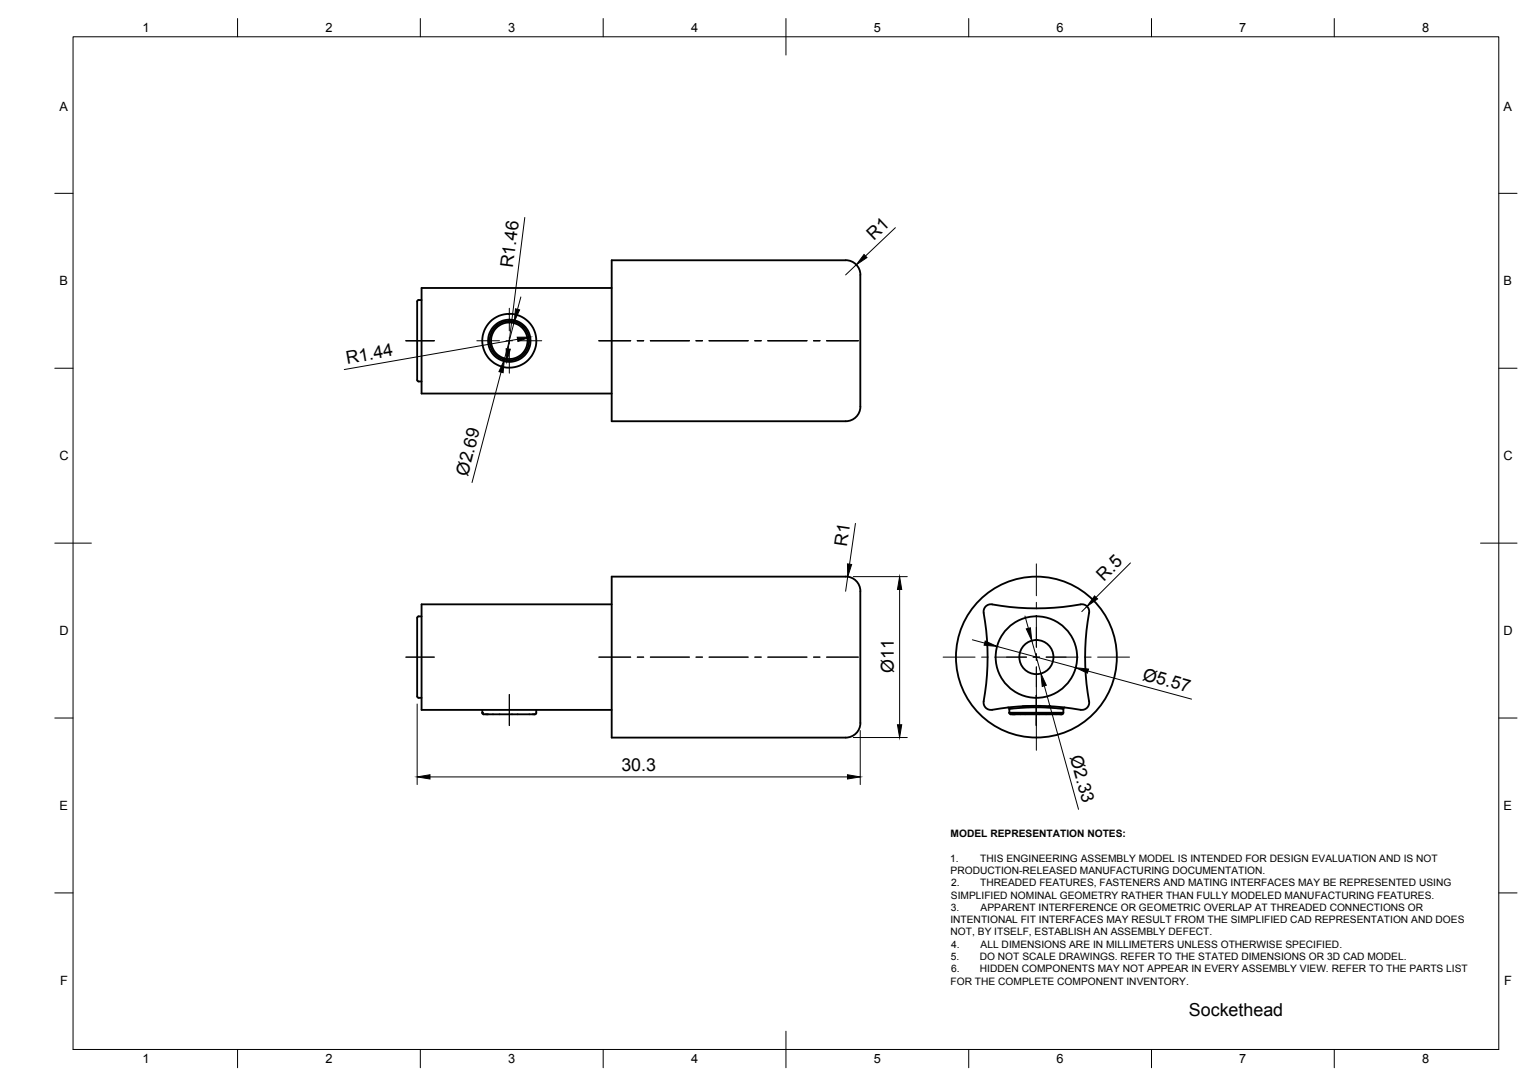
ISO-10303-21;
HEADER;
/* Generated by software containing ST-Developer
 * from STEP Tools, Inc. (www.steptools.com) 
 */

FILE_DESCRIPTION(
/* description */ ('STEP AP242 Edition 2'),
/* implementation_level */ '2;1');

FILE_NAME(
/* name */ 'Sockethead.step',
/* time_stamp */ '2026-10-06T10:11:12-07:00',
/* author */ (''),
/* organization */ (''),
/* preprocessor_version */ 'ST-DEVELOPER v20.2',
/* originating_system */ 'Autodesk Translation Framework v15.15.0.0',
/* authorisation */ '');

FILE_SCHEMA (('AUTOMOTIVE_DESIGN { 1 0 10303 214 3 1 1 }'));
ENDSEC;

DATA;
#10=MECHANICAL_DESIGN_GEOMETRIC_PRESENTATION_REPRESENTATION('',(#1787,#1788,#1789,#1790,#1791),#54580);
#235=TOROIDAL_SURFACE('',#18788,0.00268445714771808,0.0001);
#236=TOROIDAL_SURFACE('',#18804,0.00144581322131978,0.000100021493280238);
#237=TOROIDAL_SURFACE('',#18806,0.00106635989804114,0.0001);
#238=TOROIDAL_SURFACE('',#18808,0.00126635989804114,0.0001);
#239=TOROIDAL_SURFACE('',#18810,0.0045,0.001);
#1314=B_SPLINE_CURVE_WITH_KNOTS('',3,(#47239,#47240,#47241,#47242,#47243,
#47244,#47245,#47246,#47247,#47248,#47249),.UNSPECIFIED.,.F.,.F.,(4,1,1,
1,1,1,1,1,4),(3.17007800203674E-7,0.00137241382077849,0.00274482764155697,
0.00411724146233546,0.00548965528311394,0.00686206910389242,0.00823448292467091,
0.00960689674544939,0.0108038290876045),.UNSPECIFIED.);
#1315=B_SPLINE_CURVE_WITH_KNOTS('',3,(#47255,#47256,#47257,#47258,#47259,
#47260,#47261,#47262,#47263,#47264,#47265,#47266,#47267,#47268,#47269,#47270),
 .UNSPECIFIED.,.F.,.F.,(4,3,3,3,3,4),(0.5,0.51594481978154,0.641195140394408,
0.766134114390843,0.890913197743559,1.),.UNSPECIFIED.);
#1316=B_SPLINE_CURVE_WITH_KNOTS('',3,(#47271,#47272,#47273,#47274,#47275,
#47276,#47277,#47278,#47279,#47280,#47281,#47282,#47283),.UNSPECIFIED.,
 .F.,.F.,(4,3,3,3,4),(0.01606865131382,0.141192218026199,0.265882467388624,
0.390722415283828,0.5),.UNSPECIFIED.);
#1317=B_SPLINE_CURVE_WITH_KNOTS('',3,(#47323,#47324,#47325,#47326,#47327,
#47328,#47329,#47330,#47331,#47332,#47333,#47334,#47335),.UNSPECIFIED.,
 .F.,.F.,(4,3,3,3,4),(0.844373201093006,0.868421052636719,0.901315789477539,
0.934210526318359,0.956585831262424),.UNSPECIFIED.);
#1318=B_SPLINE_CURVE_WITH_KNOTS('',3,(#47337,#47338,#47339,#47340,#47341,
#47342,#47343,#47344,#47345,#47346,#47347,#47348,#47349,#47350,#47351,#47352,
#47353,#47354,#47355,#47356,#47357,#47358),.UNSPECIFIED.,.F.,.F.,(4,3,3,
3,3,3,3,4),(0.595152011141008,0.6184210546875,0.649671054199219,0.680921053710937,
0.743421052734375,0.774671052709961,0.805921052685547,0.844373201093006),
 .UNSPECIFIED.);
#1319=B_SPLINE_CURVE_WITH_KNOTS('',3,(#47360,#47361,#47362,#47363,#47364,
#47365,#47366,#47367,#47368,#47369),.UNSPECIFIED.,.F.,.F.,(4,3,3,4),(0.499571204578003,
0.524671083984375,0.55592107421875,0.595152011141008),.UNSPECIFIED.);
#1320=B_SPLINE_CURVE_WITH_KNOTS('',3,(#47371,#47372,#47373,#47374,#47375,
#47376,#47377,#47378,#47379,#47380,#47381,#47382,#47383,#47384,#47385,#47386),
 .UNSPECIFIED.,.F.,.F.,(4,3,3,3,3,4),(0.344377029418945,0.368421875,0.3996716796875,
0.430921484375,0.49342109375,0.499571204578003),.UNSPECIFIED.);
#1321=B_SPLINE_CURVE_WITH_KNOTS('',3,(#47388,#47389,#47390,#47391,#47392,
#47393,#47394,#47395,#47396,#47397,#47398,#47399,#47400,#47401,#47402,#47403,
#47404,#47405,#47406,#47407,#47408,#47409),.UNSPECIFIED.,.F.,.F.,(4,3,3,
3,3,3,3,4),(0.0951513536663715,0.11875,0.149921875,0.18109375,0.2434375,
0.27468359375,0.3059296875,0.344377029418945),.UNSPECIFIED.);
#1322=B_SPLINE_CURVE_WITH_KNOTS('',3,(#47411,#47412,#47413,#47414,#47415,
#47416,#47417),.UNSPECIFIED.,.F.,.F.,(4,3,4),(0.,0.059375,0.0951513536663715),
 .UNSPECIFIED.);
#1323=B_SPLINE_CURVE_WITH_KNOTS('',3,(#47422,#47423,#47424,#47425,#47426,
#47427,#47428,#47429,#47430,#47431,#47432,#47433,#47434,#47435,#47436,#47437,
#47438,#47439,#47440,#47441,#47442,#47443,#47444,#47445,#47446,#47447,#47448,
#47449),.UNSPECIFIED.,.F.,.F.,(4,3,3,3,3,3,3,3,3,4),(0.000439637419233018,
0.00197475622652821,0.00351361546357811,0.00505249384731604,0.00658820808674074,
0.00812412382728726,0.00966469812314125,0.0112015348521649,0.0122952440085163,
0.0122953616167891),.UNSPECIFIED.);
#1324=B_SPLINE_CURVE_WITH_KNOTS('',3,(#47498,#47499,#47500,#47501,#47502,
#47503,#47504,#47505,#47506,#47507,#47508,#47509,#47510,#47511,#47512,#47513,
#47514,#47515),.UNSPECIFIED.,.F.,.F.,(4,2,2,2,2,2,2,2,4),(0.0531545443972438,
0.0539804531362699,0.0553833366067717,0.063256430848433,0.0837219286225868,
0.0893954400242927,0.0917963407013744,0.109557936372639,0.132545890778438),
 .UNSPECIFIED.);
#1325=B_SPLINE_CURVE_WITH_KNOTS('',3,(#47519,#47520,#47521,#47522,#47523,
#47524,#47525,#47526,#47527,#47528,#47529,#47530,#47531,#47532,#47533,#47534,
#47535,#47536,#47537,#47538),.UNSPECIFIED.,.F.,.F.,(4,2,2,2,2,2,2,2,2,4),
(-0.158319955435896,-0.133815137850197,-0.106658138126813,-0.1025999008806,
-0.10032932226052,-0.0927408284757264,-0.079200925255067,-0.0410108789329117,
-0.0204087370161667,-3.15727931039809E-5),.UNSPECIFIED.);
#1326=B_SPLINE_CURVE_WITH_KNOTS('',3,(#47540,#47541,#47542,#47543,#47544,
#47545,#47546,#47547,#47548,#47549,#47550,#47551,#47552,#47553,#47554,#47555,
#47556,#47557,#47558,#47559,#47560,#47561,#47562,#47563,#47564,#47565,#47566,
#47567),.UNSPECIFIED.,.F.,.F.,(4,2,2,2,2,2,2,2,2,2,2,2,2,4),(-0.159255089654321,
-0.157276407559694,-0.15499281392426,-0.150445878334476,-0.141416102996633,
-0.123174516039657,-0.120748346467183,-0.118169256846349,-0.110388837257784,
-0.0973026115125197,-0.0773140984503772,-0.0425520341965917,-0.0212391987124548,
-0.00028544784231343),.UNSPECIFIED.);
#1327=B_SPLINE_CURVE_WITH_KNOTS('',3,(#47569,#47570,#47571,#47572,#47573,
#47574,#47575,#47576,#47577,#47578,#47579,#47580,#47581,#47582,#47583,#47584,
#47585,#47586,#47587,#47588,#47589,#47590,#47591,#47592,#47593,#47594,#47595,
#47596,#47597,#47598),.UNSPECIFIED.,.F.,.F.,(4,2,2,2,2,2,2,2,2,2,2,2,2,
2,4),(-0.159252699730232,-0.138336557138345,-0.117015600794963,-0.0822235719847124,
-0.0627557354776325,-0.0495418275572358,-0.0416948308426409,-0.0390988462294192,
-0.0341970288432549,-0.0170804313544768,-0.00858037755543813,-0.00430003517675335,
-0.00215149799157384,-0.00107591423944001,-0.000284742483905729),
 .UNSPECIFIED.);
#1328=B_SPLINE_CURVE_WITH_KNOTS('',3,(#47600,#47601,#47602,#47603,#47604,
#47605,#47606,#47607,#47608,#47609,#47610,#47611,#47612,#47613,#47614,#47615,
#47616,#47617,#47618,#47619,#47620,#47621),.UNSPECIFIED.,.F.,.F.,(4,2,2,
2,2,2,2,2,2,2,4),(-0.158572104573442,-0.138210910124321,-0.117619222785882,
-0.0794253157638306,-0.0659793598497864,-0.0584299861442276,-0.0561593995498526,
-0.0551566920948119,-0.0533519008406549,-0.0276603098885798,-0.000285004372809575),
 .UNSPECIFIED.);
#1329=B_SPLINE_CURVE_WITH_KNOTS('',3,(#47629,#47630,#47631,#47632),
 .UNSPECIFIED.,.F.,.F.,(4,4),(0.00694070085523101,0.00719068424449337),
 .UNSPECIFIED.);
#1330=B_SPLINE_CURVE_WITH_KNOTS('',3,(#47634,#47635,#47636,#47637,#47638,
#47639,#47640),.UNSPECIFIED.,.F.,.F.,(4,3,4),(0.00495768279518325,0.00594874941015533,
0.00694020764518122),.UNSPECIFIED.);
#1331=B_SPLINE_CURVE_WITH_KNOTS('',3,(#47642,#47643,#47644,#47645),
 .UNSPECIFIED.,.F.,.F.,(4,4),(0.00396583294010356,0.00495729117512944),
 .UNSPECIFIED.);
#1332=B_SPLINE_CURVE_WITH_KNOTS('',3,(#47647,#47648,#47649,#47650),
 .UNSPECIFIED.,.F.,.F.,(4,4),(0.00297486717136914,0.00396583294010356),
 .UNSPECIFIED.);
#1333=B_SPLINE_CURVE_WITH_KNOTS('',3,(#47652,#47653,#47654,#47655,#47656,
#47657,#47658),.UNSPECIFIED.,.F.,.F.,(4,3,4),(0.000991836196938153,0.00198291647005178,
0.00297437470507767),.UNSPECIFIED.);
#1334=B_SPLINE_CURVE_WITH_KNOTS('',3,(#47659,#47660,#47661,#47662),
 .UNSPECIFIED.,.F.,.F.,(4,4),(0.,0.000991458235025889),.UNSPECIFIED.);
#1335=B_SPLINE_CURVE_WITH_KNOTS('',3,(#47714,#47715,#47716,#47717),
 .UNSPECIFIED.,.F.,.F.,(4,4),(1.17608272849176E-7,0.000439637419233018),
 .UNSPECIFIED.);
#1336=B_SPLINE_CURVE_WITH_KNOTS('',3,(#47752,#47753,#47754,#47755),
 .UNSPECIFIED.,.F.,.F.,(4,4),(0.,0.01606865131382),.UNSPECIFIED.);
#1337=B_SPLINE_CURVE_WITH_KNOTS('',3,(#47756,#47757,#47758,#47759,#47760,
#47761,#47762),.UNSPECIFIED.,.F.,.F.,(4,3,4),(0.956585831262424,0.96710526315918,
1.),.UNSPECIFIED.);
#1338=B_SPLINE_CURVE_WITH_KNOTS('',3,(#47769,#47770,#47771,#47772,#47773,
#47774,#47775,#47776,#47777,#47778,#47779,#47780),.UNSPECIFIED.,.F.,.F.,
(4,2,2,2,2,4),(5.52024392907501E-5,0.0144625442992462,0.0165414513429709,
0.0327826202138422,0.0527118689517175,0.0531545443972438),.UNSPECIFIED.);
#1339=B_SPLINE_CURVE_WITH_KNOTS('',3,(#47785,#47786,#47787,#47788),
 .UNSPECIFIED.,.F.,.F.,(4,4),(8.74111736584338E-18,3.17007800203674E-7),
 .UNSPECIFIED.);
#1340=B_SPLINE_CURVE_WITH_KNOTS('',3,(#47789,#47790,#47791,#47792),
 .UNSPECIFIED.,.F.,.F.,(4,4),(0.0108038290876045,0.0109793105662279),
 .UNSPECIFIED.);
#1341=B_SPLINE_CURVE_WITH_KNOTS('',3,(#47795,#47796,#47797,#47798,#47799,
#47800,#47801),.UNSPECIFIED.,.F.,.F.,(4,3,4),(0.,0.059375,0.12171875),
 .UNSPECIFIED.);
#1342=B_SPLINE_CURVE_WITH_KNOTS('',3,(#47803,#47804,#47805,#47806,#47807,
#47808,#47809,#47810,#47811,#47812,#47813,#47814,#47815,#47816,#47817,#47818,
#47819,#47820,#47821),.UNSPECIFIED.,.F.,.F.,(4,3,3,3,3,3,4),(0.12171875,
0.1545234375,0.185851171875,0.21710505859375,0.248355252929687,0.309292762646484,
0.371714638132324),.UNSPECIFIED.);
#1343=B_SPLINE_CURVE_WITH_KNOTS('',3,(#47823,#47824,#47825,#47826,#47827,
#47828,#47829,#47830,#47831,#47832),.UNSPECIFIED.,.F.,.F.,(4,3,3,4),(0.371714638132324,
0.434210731906616,0.496710536595331,0.500091425325073),.UNSPECIFIED.);
#1344=B_SPLINE_CURVE_WITH_KNOTS('',3,(#47834,#47835,#47836,#47837,#47838,
#47839,#47840),.UNSPECIFIED.,.F.,.F.,(4,3,4),(0.500091425325073,0.559210526829766,
0.621710526341488),.UNSPECIFIED.);
#1345=B_SPLINE_CURVE_WITH_KNOTS('',3,(#47842,#47843,#47844,#47845,#47846,
#47847,#47848,#47849,#47850,#47851,#47852,#47853,#47854,#47855,#47856,#47857,
#47858,#47859,#47860),.UNSPECIFIED.,.F.,.F.,(4,3,3,3,3,3,4),(0.621710526341488,
0.684210526317074,0.746710526315854,0.779523026315793,0.81085115131579,
0.842105057565789,0.873355252878289),.UNSPECIFIED.);
#1346=B_SPLINE_CURVE_WITH_KNOTS('',3,(#47861,#47862,#47863,#47864,#47865,
#47866,#47867),.UNSPECIFIED.,.F.,.F.,(4,3,4),(0.873355252878289,0.934292762643914,
1.),.UNSPECIFIED.);
#1347=B_SPLINE_CURVE_WITH_KNOTS('',3,(#47873,#47874,#47875,#47876),
 .UNSPECIFIED.,.F.,.F.,(4,4),(0.00719068424449337,0.00793166588020711),
 .UNSPECIFIED.);
#1514=(
BOUNDED_CURVE()
B_SPLINE_CURVE(2,(#47235,#47236,#47237),.UNSPECIFIED.,.F.,.F.)
B_SPLINE_CURVE_WITH_KNOTS((3,3),(-0.999702996074256,0.),.UNSPECIFIED.)
CURVE()
GEOMETRIC_REPRESENTATION_ITEM()
RATIONAL_B_SPLINE_CURVE((0.999826070801379,0.707193771622355,1.))
REPRESENTATION_ITEM('')
);
#1515=(
BOUNDED_CURVE()
B_SPLINE_CURVE(2,(#47251,#47252,#47253),.UNSPECIFIED.,.F.,.F.)
B_SPLINE_CURVE_WITH_KNOTS((3,3),(-0.994986770849844,0.),.UNSPECIFIED.)
CURVE()
GEOMETRIC_REPRESENTATION_ITEM()
RATIONAL_B_SPLINE_CURVE((0.997078040613149,0.708575122008982,1.))
REPRESENTATION_ITEM('')
);
#1516=(
BOUNDED_CURVE()
B_SPLINE_CURVE(2,(#47319,#47320,#47321),.UNSPECIFIED.,.F.,.F.)
B_SPLINE_CURVE_WITH_KNOTS((3,3),(0.00740039126125963,1.),.UNSPECIFIED.)
CURVE()
GEOMETRIC_REPRESENTATION_ITEM()
RATIONAL_B_SPLINE_CURVE((0.995114090594777,0.669888440169379,1.))
REPRESENTATION_ITEM('')
);
#1517=(
BOUNDED_CURVE()
B_SPLINE_CURVE(2,(#47419,#47420,#47421),.UNSPECIFIED.,.F.,.F.)
B_SPLINE_CURVE_WITH_KNOTS((3,3),(-0.00697045907981074,0.999910955807272),
 .UNSPECIFIED.)
CURVE()
GEOMETRIC_REPRESENTATION_ITEM()
RATIONAL_B_SPLINE_CURVE((1.00469261537463,0.6634228407113,0.999940474400924))
REPRESENTATION_ITEM('')
);
#1518=(
BOUNDED_CURVE()
B_SPLINE_CURVE(2,(#47494,#47495,#47496),.UNSPECIFIED.,.F.,.F.)
B_SPLINE_CURVE_WITH_KNOTS((3,3),(-1.02488087602095,0.),.UNSPECIFIED.)
CURVE()
GEOMETRIC_REPRESENTATION_ITEM()
RATIONAL_B_SPLINE_CURVE((1.01354104029,0.727882565738598,1.))
REPRESENTATION_ITEM('')
);
#1519=(
BOUNDED_CURVE()
B_SPLINE_CURVE(2,(#47625,#47626,#47627),.UNSPECIFIED.,.F.,.F.)
B_SPLINE_CURVE_WITH_KNOTS((3,3),(-1.01384567949804,0.),.UNSPECIFIED.)
CURVE()
GEOMETRIC_REPRESENTATION_ITEM()
RATIONAL_B_SPLINE_CURVE((1.00769298321285,0.722188311019934,1.))
REPRESENTATION_ITEM('')
);
#1701=(
BOUNDED_SURFACE()
B_SPLINE_SURFACE(3,2,((#47200,#47201,#47202),(#47203,#47204,#47205),(#47206,
#47207,#47208),(#47209,#47210,#47211),(#47212,#47213,#47214),(#47215,#47216,
#47217),(#47218,#47219,#47220),(#47221,#47222,#47223),(#47224,#47225,#47226),
(#47227,#47228,#47229),(#47230,#47231,#47232)),.UNSPECIFIED.,.T.,.F.,.F.)
B_SPLINE_SURFACE_WITH_KNOTS((4,1,1,1,1,1,1,1,4),(3,3),(-0.0108993956052043,
-0.00953697115455376,-0.00817454670390322,-0.00681212225325268,-0.00544969780260214,
-0.0040872733519516,-0.00272484890130105,-0.00136242445065051,0.),(0.,1.00123227863135),
 .UNSPECIFIED.)
GEOMETRIC_REPRESENTATION_ITEM()
RATIONAL_B_SPLINE_SURFACE(((1.,0.706745855131733,1.00072274163255),(1.,
0.706745855131732,1.00072274163255),(1.,0.706745855131736,1.00072274163255),
(1.,0.706745855131741,1.00072274163255),(1.,0.706745855131734,1.00072274163255),
(1.,0.70674585513174,1.00072274163255),(1.,0.706745855131737,1.00072274163255),
(1.,0.706745855131739,1.00072274163255),(1.,0.706745855131743,1.00072274163255),
(1.,0.706745855131734,1.00072274163255),(1.,0.706745855131733,1.00072274163255)))
REPRESENTATION_ITEM('')
SURFACE()
);
#1702=(
BOUNDED_SURFACE()
B_SPLINE_SURFACE(3,2,((#47284,#47285,#47286),(#47287,#47288,#47289),(#47290,
#47291,#47292),(#47293,#47294,#47295),(#47296,#47297,#47298),(#47299,#47300,
#47301),(#47302,#47303,#47304),(#47305,#47306,#47307),(#47308,#47309,#47310),
(#47311,#47312,#47313),(#47314,#47315,#47316)),.UNSPECIFIED.,.T.,.F.,.F.)
B_SPLINE_SURFACE_WITH_KNOTS((4,1,1,1,1,1,1,1,4),(3,3),(-0.0121528522847183,
-0.0106337457491285,-0.00911463921353872,-0.00759553267794892,-0.00607642614235913,
-0.00455731960676934,-0.00303821307117955,-0.0015191065355898,0.),(-0.0120606504638825,
1.),.UNSPECIFIED.)
GEOMETRIC_REPRESENTATION_ITEM()
RATIONAL_B_SPLINE_SURFACE(((1.00811883844143,0.663416228430369,1.),(1.00823064312136,
0.658781126855077,1.),(1.0079877964772,0.668848852675098,1.),(1.00697574646344,
0.710805545508091,1.),(1.00731608298849,0.696696168652019,1.),(1.0083525815378,
0.653725909609466,1.),(1.00798713623623,0.668876224373087,1.),(1.00697515363204,
0.710830122598659,1.),(1.00731696839763,0.696659462126846,1.),(1.0080070337615,
0.66805133000566,1.),(1.00811883844143,0.663416228430369,1.)))
REPRESENTATION_ITEM('')
SURFACE()
);
#1703=(
BOUNDED_SURFACE()
B_SPLINE_SURFACE(3,2,((#47450,#47451,#47452),(#47453,#47454,#47455),(#47456,
#47457,#47458),(#47459,#47460,#47461),(#47462,#47463,#47464),(#47465,#47466,
#47467),(#47468,#47469,#47470),(#47471,#47472,#47473),(#47474,#47475,#47476),
(#47477,#47478,#47479),(#47480,#47481,#47482),(#47483,#47484,#47485),(#47486,
#47487,#47488),(#47489,#47490,#47491)),.UNSPECIFIED.,.T.,.F.,.F.)
B_SPLINE_SURFACE_WITH_KNOTS((4,1,1,1,1,1,1,1,3,4),(3,3),(-0.00765457458290781,
-0.00738843513850202,-0.00633294440443031,-0.00527745367035859,-0.00422196293628687,
-0.00316647220221515,-0.00211098146814344,-0.00105549073407172,0.,0.000789351289665934),
(0.,1.05454521855088),.UNSPECIFIED.)
GEOMETRIC_REPRESENTATION_ITEM()
RATIONAL_B_SPLINE_SURFACE(((1.,0.711036106532509,1.03152319744499),(1.,
0.709345031579044,1.03170767755084),(1.,0.70035057317659,1.03268888694945),
(1.,0.683782910015655,1.03449626056544),(1.,0.705801584459776,1.03209423374593),
(1.,0.727101128800789,1.0297706571437),(1.,0.705831990732036,1.03209091671239),
(1.,0.683783260356914,1.03449622234655),(1.,0.705820110962035,1.0320922126817),
(1.,0.720001022829777,1.03054521080754),(1.,0.720006348153552,1.03054462986564),
(1.,0.720010330709774,1.03054419540685),(1.,0.716051718549058,1.03097604213777),
(1.,0.711036106532509,1.03152319744499)))
REPRESENTATION_ITEM('')
SURFACE()
);
#1704=(
BOUNDED_SURFACE()
B_SPLINE_SURFACE(3,2,((#47877,#47878,#47879),(#47880,#47881,#47882),(#47883,
#47884,#47885),(#47886,#47887,#47888),(#47889,#47890,#47891),(#47892,#47893,
#47894),(#47895,#47896,#47897),(#47898,#47899,#47900),(#47901,#47902,#47903),
(#47904,#47905,#47906),(#47907,#47908,#47909)),.UNSPECIFIED.,.T.,.F.,.F.)
B_SPLINE_SURFACE_WITH_KNOTS((4,1,1,1,1,1,1,1,4),(3,3),(0.,0.00105549073407172,
0.00211098146814343,0.00316647220221515,0.00422196293628687,0.00527745367035859,
0.0063329444044303,0.00738843513850202,0.00844392587257374),(0.,1.05454521855088),
 .UNSPECIFIED.)
GEOMETRIC_REPRESENTATION_ITEM()
RATIONAL_B_SPLINE_SURFACE(((1.,0.720006348153552,1.03054462986564),(1.,
0.720011673477327,1.03054404892375),(1.,0.705852062904688,1.03208872703031),
(1.,0.683782910015655,1.03449626056544),(1.,0.705801584459776,1.03209423374593),
(1.,0.727101128800789,1.0297706571437),(1.,0.705831990732036,1.03209091671239),
(1.,0.683783260356914,1.03449622234655),(1.,0.705820110962035,1.0320922126817),
(1.,0.720001022829777,1.03054521080754),(1.,0.720006348153552,1.03054462986564)))
REPRESENTATION_ITEM('')
SURFACE()
);
#1705=(
BOUNDED_SURFACE()
B_SPLINE_SURFACE(3,2,((#47910,#47911,#47912),(#47913,#47914,#47915),(#47916,
#47917,#47918),(#47919,#47920,#47921),(#47922,#47923,#47924),(#47925,#47926,
#47927),(#47928,#47929,#47930),(#47931,#47932,#47933),(#47934,#47935,#47936),
(#47937,#47938,#47939),(#47940,#47941,#47942)),.UNSPECIFIED.,.T.,.F.,.F.)
B_SPLINE_SURFACE_WITH_KNOTS((4,1,1,1,1,1,1,1,4),(3,3),(0.,0.00151910653558979,
0.00303821307117958,0.00455731960676938,0.00607642614235917,0.00759553267794896,
0.00911463921353875,0.0106337457491285,0.0121528522847183),(-0.0120606504638825,
1.),.UNSPECIFIED.)
GEOMETRIC_REPRESENTATION_ITEM()
RATIONAL_B_SPLINE_SURFACE(((1.00811883844143,0.663416228430369,1.),(1.00823064312136,
0.658781126855077,1.),(1.0079877964772,0.668848852675098,1.),(1.00697574646344,
0.710805545508091,1.),(1.00731608298849,0.696696168652019,1.),(1.0083525815378,
0.653725909609466,1.),(1.00798713623623,0.668876224373087,1.),(1.00697515363204,
0.710830122598659,1.),(1.00731696839763,0.696659462126846,1.),(1.0080070337615,
0.66805133000566,1.),(1.00811883844143,0.663416228430369,1.)))
REPRESENTATION_ITEM('')
SURFACE()
);
#1706=(
BOUNDED_SURFACE()
B_SPLINE_SURFACE(3,2,((#47945,#47946,#47947),(#47948,#47949,#47950),(#47951,
#47952,#47953),(#47954,#47955,#47956),(#47957,#47958,#47959),(#47960,#47961,
#47962),(#47963,#47964,#47965),(#47966,#47967,#47968),(#47969,#47970,#47971),
(#47972,#47973,#47974),(#47975,#47976,#47977)),.UNSPECIFIED.,.T.,.F.,.F.)
B_SPLINE_SURFACE_WITH_KNOTS((4,1,1,1,1,1,1,1,4),(3,3),(0.,0.00136242445065054,
0.00272484890130108,0.00408727335195162,0.00544969780260216,0.0068121222532527,
0.00817454670390325,0.00953697115455379,0.0108993956052043),(0.,1.00123227863135),
 .UNSPECIFIED.)
GEOMETRIC_REPRESENTATION_ITEM()
RATIONAL_B_SPLINE_SURFACE(((1.,0.706745855131733,1.00072274163255),(1.,
0.706745855131732,1.00072274163255),(1.,0.706745855131736,1.00072274163255),
(1.,0.706745855131741,1.00072274163255),(1.,0.706745855131734,1.00072274163255),
(1.,0.70674585513174,1.00072274163255),(1.,0.706745855131737,1.00072274163255),
(1.,0.706745855131739,1.00072274163255),(1.,0.706745855131743,1.00072274163255),
(1.,0.706745855131734,1.00072274163255),(1.,0.706745855131733,1.00072274163255)))
REPRESENTATION_ITEM('')
SURFACE()
);
#1747=SHAPE_REPRESENTATION_RELATIONSHIP('SRR','None',#54634,#1761);
#1761=ADVANCED_BREP_SHAPE_REPRESENTATION('',(#1805),#54570);
#1787=STYLED_ITEM('',(#54715),#17257);
#1788=STYLED_ITEM('',(#54713),#17258);
#1789=STYLED_ITEM('',(#54713),#17272);
#1790=STYLED_ITEM('',(#54713),#17284);
#1791=STYLED_ITEM('',(#54709),#1805);
#1805=MANIFOLD_SOLID_BREP('Body1',#17670);
#2087=LINE('',#47685,#2680);
#2088=LINE('',#47709,#2681);
#2089=LINE('',#47710,#2682);
#2090=LINE('',#47712,#2683);
#2091=LINE('',#47713,#2684);
#2092=LINE('',#47719,#2685);
#2093=LINE('',#47720,#2686);
#2094=LINE('',#47722,#2687);
#2095=LINE('',#47723,#2688);
#2096=LINE('',#47730,#2689);
#2097=LINE('',#47745,#2690);
#2098=LINE('',#47751,#2691);
#2099=LINE('',#47767,#2692);
#2100=LINE('',#47872,#2693);
#2680=VECTOR('',#21727,0.0055);
#2681=VECTOR('',#21754,1.);
#2682=VECTOR('',#21755,1.);
#2683=VECTOR('',#21758,1.);
#2684=VECTOR('',#21759,1.);
#2685=VECTOR('',#21762,1.);
#2686=VECTOR('',#21763,1.);
#2687=VECTOR('',#21766,1.);
#2688=VECTOR('',#21767,1.);
#2689=VECTOR('',#21778,0.00278445714771807);
#2690=VECTOR('',#21797,0.00116635989804114);
#2691=VECTOR('',#21806,0.00184479343283513);
#2692=VECTOR('',#21811,0.00134583534834952);
#2693=VECTOR('',#21824,0.00125);
#3315=CYLINDRICAL_SURFACE('',#18760,0.0055);
#3316=CYLINDRICAL_SURFACE('',#18774,0.017);
#3317=CYLINDRICAL_SURFACE('',#18775,0.017);
#3318=CYLINDRICAL_SURFACE('',#18776,0.017);
#3319=CYLINDRICAL_SURFACE('',#18777,0.017);
#3320=CYLINDRICAL_SURFACE('',#18778,0.0005);
#3321=CYLINDRICAL_SURFACE('',#18779,0.0005);
#3322=CYLINDRICAL_SURFACE('',#18780,0.0005);
#3323=CYLINDRICAL_SURFACE('',#18781,0.0005);
#3324=CYLINDRICAL_SURFACE('',#18782,0.00278445714771807);
#3325=CYLINDRICAL_SURFACE('',#18790,0.00116635989804114);
#3326=CYLINDRICAL_SURFACE('',#18795,0.00184479343283513);
#3327=CYLINDRICAL_SURFACE('',#18796,0.00134583534834952);
#3328=CYLINDRICAL_SURFACE('',#18803,0.00125);
#3501=FACE_BOUND('',#5171,.T.);
#3502=FACE_BOUND('',#5175,.T.);
#3503=FACE_BOUND('',#5178,.T.);
#3504=FACE_BOUND('',#5187,.T.);
#3505=FACE_BOUND('',#5194,.T.);
#4137=FACE_OUTER_BOUND('',#5167,.T.);
#4138=FACE_OUTER_BOUND('',#5168,.T.);
#4139=FACE_OUTER_BOUND('',#5169,.T.);
#4140=FACE_OUTER_BOUND('',#5170,.T.);
#4141=FACE_OUTER_BOUND('',#5172,.T.);
#4142=FACE_OUTER_BOUND('',#5173,.T.);
#4143=FACE_OUTER_BOUND('',#5174,.T.);
#4144=FACE_OUTER_BOUND('',#5176,.T.);
#4145=FACE_OUTER_BOUND('',#5177,.T.);
#4146=FACE_OUTER_BOUND('',#5179,.T.);
#4147=FACE_OUTER_BOUND('',#5180,.T.);
#4148=FACE_OUTER_BOUND('',#5181,.T.);
#4149=FACE_OUTER_BOUND('',#5182,.T.);
#4150=FACE_OUTER_BOUND('',#5183,.T.);
#4151=FACE_OUTER_BOUND('',#5184,.T.);
#4152=FACE_OUTER_BOUND('',#5185,.T.);
#4153=FACE_OUTER_BOUND('',#5186,.T.);
#4154=FACE_OUTER_BOUND('',#5188,.T.);
#4155=FACE_OUTER_BOUND('',#5189,.T.);
#4156=FACE_OUTER_BOUND('',#5190,.T.);
#4157=FACE_OUTER_BOUND('',#5191,.T.);
#4158=FACE_OUTER_BOUND('',#5192,.T.);
#4159=FACE_OUTER_BOUND('',#5193,.T.);
#4160=FACE_OUTER_BOUND('',#5195,.T.);
#4161=FACE_OUTER_BOUND('',#5196,.T.);
#4162=FACE_OUTER_BOUND('',#5197,.T.);
#4163=FACE_OUTER_BOUND('',#5198,.T.);
#4164=FACE_OUTER_BOUND('',#5199,.T.);
#4165=FACE_OUTER_BOUND('',#5200,.T.);
#4166=FACE_OUTER_BOUND('',#5201,.T.);
#4167=FACE_OUTER_BOUND('',#5202,.T.);
#4168=FACE_OUTER_BOUND('',#5203,.T.);
#5167=EDGE_LOOP('',(#14557,#14558,#14559,#14560,#14561));
#5168=EDGE_LOOP('',(#14562,#14563,#14564,#14565,#14566,#14567,#14568,#14569,
#14570));
#5169=EDGE_LOOP('',(#14571,#14572,#14573,#14574,#14575,#14576,#14577,#14578,
#14579,#14580,#14581,#14582,#14583,#14584,#14585));
#5170=EDGE_LOOP('',(#14586));
#5171=EDGE_LOOP('',(#14587,#14588,#14589,#14590,#14591,#14592,#14593,#14594));
#5172=EDGE_LOOP('',(#14595,#14596,#14597,#14598));
#5173=EDGE_LOOP('',(#14599));
#5174=EDGE_LOOP('',(#14600,#14601,#14602,#14603,#14604,#14605,#14606,#14607));
#5175=EDGE_LOOP('',(#14608));
#5176=EDGE_LOOP('',(#14609,#14610,#14611,#14612));
#5177=EDGE_LOOP('',(#14613,#14614,#14615,#14616));
#5178=EDGE_LOOP('',(#14617,#14618));
#5179=EDGE_LOOP('',(#14619,#14620,#14621,#14622));
#5180=EDGE_LOOP('',(#14623,#14624,#14625,#14626));
#5181=EDGE_LOOP('',(#14627,#14628,#14629,#14630));
#5182=EDGE_LOOP('',(#14631,#14632,#14633,#14634));
#5183=EDGE_LOOP('',(#14635,#14636,#14637,#14638));
#5184=EDGE_LOOP('',(#14639,#14640,#14641,#14642));
#5185=EDGE_LOOP('',(#14643,#14644,#14645,#14646,#14647));
#5186=EDGE_LOOP('',(#14648));
#5187=EDGE_LOOP('',(#14649));
#5188=EDGE_LOOP('',(#14650,#14651,#14652,#14653,#14654));
#5189=EDGE_LOOP('',(#14655,#14656,#14657,#14658));
#5190=EDGE_LOOP('',(#14659));
#5191=EDGE_LOOP('',(#14660,#14661,#14662,#14663,#14664,#14665,#14666,#14667,
#14668,#14669,#14670,#14671));
#5192=EDGE_LOOP('',(#14672,#14673,#14674,#14675,#14676,#14677,#14678,#14679,
#14680,#14681,#14682,#14683,#14684));
#5193=EDGE_LOOP('',(#14685,#14686,#14687));
#5194=EDGE_LOOP('',(#14688,#14689,#14690,#14691,#14692,#14693));
#5195=EDGE_LOOP('',(#14694));
#5196=EDGE_LOOP('',(#14695,#14696,#14697,#14698,#14699,#14700,#14701,#14702,
#14703,#14704));
#5197=EDGE_LOOP('',(#14705,#14706,#14707,#14708,#14709));
#5198=EDGE_LOOP('',(#14710,#14711,#14712,#14713));
#5199=EDGE_LOOP('',(#14714,#14715,#14716,#14717,#14718,#14719,#14720,#14721,
#14722,#14723));
#5200=EDGE_LOOP('',(#14724,#14725,#14726,#14727,#14728));
#5201=EDGE_LOOP('',(#14729,#14730,#14731,#14732));
#5202=EDGE_LOOP('',(#14733,#14734,#14735,#14736));
#5203=EDGE_LOOP('',(#14737,#14738,#14739,#14740));
#6121=CIRCLE('',#18748,0.00134890248414929);
#6122=CIRCLE('',#18749,0.00134890252382471);
#6123=CIRCLE('',#18751,0.0055);
#6124=CIRCLE('',#18752,0.017);
#6125=CIRCLE('',#18753,0.0005);
#6126=CIRCLE('',#18754,0.017);
#6127=CIRCLE('',#18755,0.0005);
#6128=CIRCLE('',#18756,0.017);
#6129=CIRCLE('',#18757,0.0005);
#6130=CIRCLE('',#18758,0.017);
#6131=CIRCLE('',#18759,0.0005);
#6132=CIRCLE('',#18761,0.0055);
#6133=CIRCLE('',#18763,0.0045);
#6134=CIRCLE('',#18765,0.017);
#6135=CIRCLE('',#18766,0.0005);
#6136=CIRCLE('',#18767,0.017);
#6137=CIRCLE('',#18768,0.0005);
#6138=CIRCLE('',#18769,0.017);
#6139=CIRCLE('',#18770,0.0005);
#6140=CIRCLE('',#18771,0.017);
#6141=CIRCLE('',#18772,0.0005);
#6142=CIRCLE('',#18773,0.00278445714771807);
#6143=CIRCLE('',#18783,0.00278445714771807);
#6144=CIRCLE('',#18784,0.00278445714771807);
#6145=CIRCLE('',#18786,0.00268445714771808);
#6146=CIRCLE('',#18787,0.00126635989804114);
#6147=CIRCLE('',#18789,0.0001);
#6148=CIRCLE('',#18791,0.00116635989804114);
#6149=CIRCLE('',#18792,0.00116635989804114);
#6150=CIRCLE('',#18794,0.00106635989804114);
#6151=CIRCLE('',#18797,0.00134579174568697);
#6152=CIRCLE('',#18798,0.00134832773590515);
#6153=CIRCLE('',#18799,0.00134579174568697);
#6154=CIRCLE('',#18802,0.00125);
#6155=CIRCLE('',#18805,0.000100021493280238);
#6156=CIRCLE('',#18807,0.0001);
#6157=CIRCLE('',#18809,0.0001);
#6158=CIRCLE('',#18811,0.001);
#7705=VERTEX_POINT('',#47233);
#7706=VERTEX_POINT('',#47234);
#7707=VERTEX_POINT('',#47238);
#7708=VERTEX_POINT('',#47250);
#7709=VERTEX_POINT('',#47254);
#7710=VERTEX_POINT('',#47317);
#7711=VERTEX_POINT('',#47318);
#7712=VERTEX_POINT('',#47322);
#7713=VERTEX_POINT('',#47336);
#7714=VERTEX_POINT('',#47359);
#7715=VERTEX_POINT('',#47370);
#7716=VERTEX_POINT('',#47387);
#7717=VERTEX_POINT('',#47410);
#7718=VERTEX_POINT('',#47418);
#7719=VERTEX_POINT('',#47492);
#7720=VERTEX_POINT('',#47493);
#7721=VERTEX_POINT('',#47497);
#7722=VERTEX_POINT('',#47516);
#7723=VERTEX_POINT('',#47518);
#7724=VERTEX_POINT('',#47539);
#7725=VERTEX_POINT('',#47568);
#7726=VERTEX_POINT('',#47599);
#7727=VERTEX_POINT('',#47622);
#7728=VERTEX_POINT('',#47624);
#7729=VERTEX_POINT('',#47628);
#7730=VERTEX_POINT('',#47633);
#7731=VERTEX_POINT('',#47641);
#7732=VERTEX_POINT('',#47646);
#7733=VERTEX_POINT('',#47651);
#7734=VERTEX_POINT('',#47664);
#7735=VERTEX_POINT('',#47666);
#7736=VERTEX_POINT('',#47667);
#7737=VERTEX_POINT('',#47669);
#7738=VERTEX_POINT('',#47671);
#7739=VERTEX_POINT('',#47673);
#7740=VERTEX_POINT('',#47675);
#7741=VERTEX_POINT('',#47677);
#7742=VERTEX_POINT('',#47679);
#7743=VERTEX_POINT('',#47683);
#7744=VERTEX_POINT('',#47687);
#7745=VERTEX_POINT('',#47690);
#7746=VERTEX_POINT('',#47691);
#7747=VERTEX_POINT('',#47693);
#7748=VERTEX_POINT('',#47695);
#7749=VERTEX_POINT('',#47697);
#7750=VERTEX_POINT('',#47699);
#7751=VERTEX_POINT('',#47701);
#7752=VERTEX_POINT('',#47703);
#7753=VERTEX_POINT('',#47706);
#7754=VERTEX_POINT('',#47729);
#7755=VERTEX_POINT('',#47731);
#7756=VERTEX_POINT('',#47735);
#7757=VERTEX_POINT('',#47737);
#7758=VERTEX_POINT('',#47742);
#7759=VERTEX_POINT('',#47744);
#7760=VERTEX_POINT('',#47748);
#7761=VERTEX_POINT('',#47764);
#7762=VERTEX_POINT('',#47765);
#7763=VERTEX_POINT('',#47768);
#7764=VERTEX_POINT('',#47784);
#7765=VERTEX_POINT('',#47793);
#7766=VERTEX_POINT('',#47794);
#7767=VERTEX_POINT('',#47802);
#7768=VERTEX_POINT('',#47822);
#7769=VERTEX_POINT('',#47833);
#7770=VERTEX_POINT('',#47841);
#7771=VERTEX_POINT('',#47869);
#10070=EDGE_CURVE('',#7705,#7706,#1514,.T.);
#10071=EDGE_CURVE('',#7707,#7705,#1314,.T.);
#10072=EDGE_CURVE('',#7707,#7708,#1515,.T.);
#10073=EDGE_CURVE('',#7709,#7708,#1315,.T.);
#10074=EDGE_CURVE('',#7706,#7709,#1316,.T.);
#10075=EDGE_CURVE('',#7710,#7711,#1516,.T.);
#10076=EDGE_CURVE('',#7712,#7710,#1317,.T.);
#10077=EDGE_CURVE('',#7713,#7712,#1318,.T.);
#10078=EDGE_CURVE('',#7714,#7713,#1319,.T.);
#10079=EDGE_CURVE('',#7715,#7714,#1320,.T.);
#10080=EDGE_CURVE('',#7716,#7715,#1321,.T.);
#10081=EDGE_CURVE('',#7717,#7716,#1322,.T.);
#10082=EDGE_CURVE('',#7717,#7718,#1517,.T.);
#10083=EDGE_CURVE('',#7711,#7718,#1323,.T.);
#10084=EDGE_CURVE('',#7719,#7720,#1518,.T.);
#10085=EDGE_CURVE('',#7719,#7721,#1324,.T.);
#10086=EDGE_CURVE('',#7722,#7721,#6121,.T.);
#10087=EDGE_CURVE('',#7722,#7723,#1325,.F.);
#10088=EDGE_CURVE('',#7724,#7723,#1326,.T.);
#10089=EDGE_CURVE('',#7724,#7725,#1327,.F.);
#10090=EDGE_CURVE('',#7726,#7725,#1328,.T.);
#10091=EDGE_CURVE('',#7727,#7726,#6122,.T.);
#10092=EDGE_CURVE('',#7727,#7728,#1519,.T.);
#10093=EDGE_CURVE('',#7729,#7728,#1329,.T.);
#10094=EDGE_CURVE('',#7730,#7729,#1330,.T.);
#10095=EDGE_CURVE('',#7731,#7730,#1331,.T.);
#10096=EDGE_CURVE('',#7732,#7731,#1332,.T.);
#10097=EDGE_CURVE('',#7733,#7732,#1333,.T.);
#10098=EDGE_CURVE('',#7720,#7733,#1334,.T.);
#10099=EDGE_CURVE('',#7734,#7734,#6123,.T.);
#10100=EDGE_CURVE('',#7735,#7736,#6124,.F.);
#10101=EDGE_CURVE('',#7736,#7737,#6125,.T.);
#10102=EDGE_CURVE('',#7737,#7738,#6126,.F.);
#10103=EDGE_CURVE('',#7738,#7739,#6127,.T.);
#10104=EDGE_CURVE('',#7739,#7740,#6128,.F.);
#10105=EDGE_CURVE('',#7740,#7741,#6129,.T.);
#10106=EDGE_CURVE('',#7741,#7742,#6130,.F.);
#10107=EDGE_CURVE('',#7742,#7735,#6131,.T.);
#10108=EDGE_CURVE('',#7743,#7743,#6132,.F.);
#10109=EDGE_CURVE('',#7743,#7734,#2087,.T.);
#10110=EDGE_CURVE('',#7744,#7744,#6133,.T.);
#10111=EDGE_CURVE('',#7745,#7746,#6134,.F.);
#10112=EDGE_CURVE('',#7746,#7747,#6135,.T.);
#10113=EDGE_CURVE('',#7747,#7748,#6136,.F.);
#10114=EDGE_CURVE('',#7748,#7749,#6137,.T.);
#10115=EDGE_CURVE('',#7749,#7750,#6138,.F.);
#10116=EDGE_CURVE('',#7750,#7751,#6139,.T.);
#10117=EDGE_CURVE('',#7751,#7752,#6140,.F.);
#10118=EDGE_CURVE('',#7752,#7745,#6141,.T.);
#10119=EDGE_CURVE('',#7753,#7753,#6142,.T.);
#10120=EDGE_CURVE('',#7751,#7742,#2088,.T.);
#10121=EDGE_CURVE('',#7741,#7752,#2089,.F.);
#10122=EDGE_CURVE('',#7739,#7746,#2090,.F.);
#10123=EDGE_CURVE('',#7745,#7740,#2091,.T.);
#10124=EDGE_CURVE('',#7718,#7711,#1335,.T.);
#10125=EDGE_CURVE('',#7749,#7736,#2092,.T.);
#10126=EDGE_CURVE('',#7735,#7750,#2093,.F.);
#10127=EDGE_CURVE('',#7747,#7738,#2094,.T.);
#10128=EDGE_CURVE('',#7737,#7748,#2095,.F.);
#10129=EDGE_CURVE('',#7753,#7754,#2096,.T.);
#10130=EDGE_CURVE('',#7754,#7755,#6143,.F.);
#10131=EDGE_CURVE('',#7755,#7754,#6144,.F.);
#10132=EDGE_CURVE('',#7756,#7756,#6145,.T.);
#10133=EDGE_CURVE('',#7757,#7757,#6146,.F.);
#10134=EDGE_CURVE('',#7756,#7755,#6147,.T.);
#10135=EDGE_CURVE('',#7758,#7758,#6148,.F.);
#10136=EDGE_CURVE('',#7758,#7759,#2097,.T.);
#10137=EDGE_CURVE('',#7759,#7759,#6149,.T.);
#10138=EDGE_CURVE('',#7760,#7760,#6150,.T.);
#10139=EDGE_CURVE('',#7714,#7709,#2098,.T.);
#10140=EDGE_CURVE('',#7708,#7706,#1336,.T.);
#10141=EDGE_CURVE('',#7710,#7717,#1337,.T.);
#10142=EDGE_CURVE('',#7761,#7762,#6151,.T.);
#10143=EDGE_CURVE('',#7762,#7724,#2099,.T.);
#10144=EDGE_CURVE('',#7763,#7719,#1338,.T.);
#10145=EDGE_CURVE('',#7763,#7727,#6152,.T.);
#10146=EDGE_CURVE('',#7762,#7761,#6153,.T.);
#10147=EDGE_CURVE('',#7764,#7707,#1339,.T.);
#10148=EDGE_CURVE('',#7705,#7764,#1340,.T.);
#10149=EDGE_CURVE('',#7765,#7766,#1341,.T.);
#10150=EDGE_CURVE('',#7766,#7767,#1342,.T.);
#10151=EDGE_CURVE('',#7767,#7768,#1343,.T.);
#10152=EDGE_CURVE('',#7768,#7769,#1344,.T.);
#10153=EDGE_CURVE('',#7769,#7770,#1345,.T.);
#10154=EDGE_CURVE('',#7770,#7765,#1346,.T.);
#10155=EDGE_CURVE('',#7771,#7771,#6154,.T.);
#10156=EDGE_CURVE('',#7731,#7771,#2100,.T.);
#10157=EDGE_CURVE('',#7728,#7720,#1347,.T.);
#10158=EDGE_CURVE('',#7768,#7762,#6155,.T.);
#10159=EDGE_CURVE('',#7760,#7758,#6156,.T.);
#10160=EDGE_CURVE('',#7759,#7757,#6157,.T.);
#10161=EDGE_CURVE('',#7744,#7743,#6158,.T.);
#14557=ORIENTED_EDGE('',*,*,#10070,.F.);
#14558=ORIENTED_EDGE('',*,*,#10071,.F.);
#14559=ORIENTED_EDGE('',*,*,#10072,.T.);
#14560=ORIENTED_EDGE('',*,*,#10073,.F.);
#14561=ORIENTED_EDGE('',*,*,#10074,.F.);
#14562=ORIENTED_EDGE('',*,*,#10075,.F.);
#14563=ORIENTED_EDGE('',*,*,#10076,.F.);
#14564=ORIENTED_EDGE('',*,*,#10077,.F.);
#14565=ORIENTED_EDGE('',*,*,#10078,.F.);
#14566=ORIENTED_EDGE('',*,*,#10079,.F.);
#14567=ORIENTED_EDGE('',*,*,#10080,.F.);
#14568=ORIENTED_EDGE('',*,*,#10081,.F.);
#14569=ORIENTED_EDGE('',*,*,#10082,.T.);
#14570=ORIENTED_EDGE('',*,*,#10083,.F.);
#14571=ORIENTED_EDGE('',*,*,#10084,.F.);
#14572=ORIENTED_EDGE('',*,*,#10085,.T.);
#14573=ORIENTED_EDGE('',*,*,#10086,.F.);
#14574=ORIENTED_EDGE('',*,*,#10087,.T.);
#14575=ORIENTED_EDGE('',*,*,#10088,.F.);
#14576=ORIENTED_EDGE('',*,*,#10089,.T.);
#14577=ORIENTED_EDGE('',*,*,#10090,.F.);
#14578=ORIENTED_EDGE('',*,*,#10091,.F.);
#14579=ORIENTED_EDGE('',*,*,#10092,.T.);
#14580=ORIENTED_EDGE('',*,*,#10093,.F.);
#14581=ORIENTED_EDGE('',*,*,#10094,.F.);
#14582=ORIENTED_EDGE('',*,*,#10095,.F.);
#14583=ORIENTED_EDGE('',*,*,#10096,.F.);
#14584=ORIENTED_EDGE('',*,*,#10097,.F.);
#14585=ORIENTED_EDGE('',*,*,#10098,.F.);
#14586=ORIENTED_EDGE('',*,*,#10099,.F.);
#14587=ORIENTED_EDGE('',*,*,#10100,.T.);
#14588=ORIENTED_EDGE('',*,*,#10101,.T.);
#14589=ORIENTED_EDGE('',*,*,#10102,.T.);
#14590=ORIENTED_EDGE('',*,*,#10103,.T.);
#14591=ORIENTED_EDGE('',*,*,#10104,.T.);
#14592=ORIENTED_EDGE('',*,*,#10105,.T.);
#14593=ORIENTED_EDGE('',*,*,#10106,.T.);
#14594=ORIENTED_EDGE('',*,*,#10107,.T.);
#14595=ORIENTED_EDGE('',*,*,#10108,.T.);
#14596=ORIENTED_EDGE('',*,*,#10109,.T.);
#14597=ORIENTED_EDGE('',*,*,#10099,.T.);
#14598=ORIENTED_EDGE('',*,*,#10109,.F.);
#14599=ORIENTED_EDGE('',*,*,#10110,.T.);
#14600=ORIENTED_EDGE('',*,*,#10111,.T.);
#14601=ORIENTED_EDGE('',*,*,#10112,.T.);
#14602=ORIENTED_EDGE('',*,*,#10113,.T.);
#14603=ORIENTED_EDGE('',*,*,#10114,.T.);
#14604=ORIENTED_EDGE('',*,*,#10115,.T.);
#14605=ORIENTED_EDGE('',*,*,#10116,.T.);
#14606=ORIENTED_EDGE('',*,*,#10117,.T.);
#14607=ORIENTED_EDGE('',*,*,#10118,.T.);
#14608=ORIENTED_EDGE('',*,*,#10119,.F.);
#14609=ORIENTED_EDGE('',*,*,#10117,.F.);
#14610=ORIENTED_EDGE('',*,*,#10120,.T.);
#14611=ORIENTED_EDGE('',*,*,#10106,.F.);
#14612=ORIENTED_EDGE('',*,*,#10121,.T.);
#14613=ORIENTED_EDGE('',*,*,#10104,.F.);
#14614=ORIENTED_EDGE('',*,*,#10122,.T.);
#14615=ORIENTED_EDGE('',*,*,#10111,.F.);
#14616=ORIENTED_EDGE('',*,*,#10123,.T.);
#14617=ORIENTED_EDGE('',*,*,#10124,.T.);
#14618=ORIENTED_EDGE('',*,*,#10083,.T.);
#14619=ORIENTED_EDGE('',*,*,#10115,.F.);
#14620=ORIENTED_EDGE('',*,*,#10125,.T.);
#14621=ORIENTED_EDGE('',*,*,#10100,.F.);
#14622=ORIENTED_EDGE('',*,*,#10126,.T.);
#14623=ORIENTED_EDGE('',*,*,#10113,.F.);
#14624=ORIENTED_EDGE('',*,*,#10127,.T.);
#14625=ORIENTED_EDGE('',*,*,#10102,.F.);
#14626=ORIENTED_EDGE('',*,*,#10128,.T.);
#14627=ORIENTED_EDGE('',*,*,#10112,.F.);
#14628=ORIENTED_EDGE('',*,*,#10122,.F.);
#14629=ORIENTED_EDGE('',*,*,#10103,.F.);
#14630=ORIENTED_EDGE('',*,*,#10127,.F.);
#14631=ORIENTED_EDGE('',*,*,#10114,.F.);
#14632=ORIENTED_EDGE('',*,*,#10128,.F.);
#14633=ORIENTED_EDGE('',*,*,#10101,.F.);
#14634=ORIENTED_EDGE('',*,*,#10125,.F.);
#14635=ORIENTED_EDGE('',*,*,#10116,.F.);
#14636=ORIENTED_EDGE('',*,*,#10126,.F.);
#14637=ORIENTED_EDGE('',*,*,#10107,.F.);
#14638=ORIENTED_EDGE('',*,*,#10120,.F.);
#14639=ORIENTED_EDGE('',*,*,#10118,.F.);
#14640=ORIENTED_EDGE('',*,*,#10121,.F.);
#14641=ORIENTED_EDGE('',*,*,#10105,.F.);
#14642=ORIENTED_EDGE('',*,*,#10123,.F.);
#14643=ORIENTED_EDGE('',*,*,#10119,.T.);
#14644=ORIENTED_EDGE('',*,*,#10129,.T.);
#14645=ORIENTED_EDGE('',*,*,#10130,.T.);
#14646=ORIENTED_EDGE('',*,*,#10131,.T.);
#14647=ORIENTED_EDGE('',*,*,#10129,.F.);
#14648=ORIENTED_EDGE('',*,*,#10132,.T.);
#14649=ORIENTED_EDGE('',*,*,#10133,.T.);
#14650=ORIENTED_EDGE('',*,*,#10132,.F.);
#14651=ORIENTED_EDGE('',*,*,#10134,.T.);
#14652=ORIENTED_EDGE('',*,*,#10130,.F.);
#14653=ORIENTED_EDGE('',*,*,#10131,.F.);
#14654=ORIENTED_EDGE('',*,*,#10134,.F.);
#14655=ORIENTED_EDGE('',*,*,#10135,.T.);
#14656=ORIENTED_EDGE('',*,*,#10136,.T.);
#14657=ORIENTED_EDGE('',*,*,#10137,.T.);
#14658=ORIENTED_EDGE('',*,*,#10136,.F.);
#14659=ORIENTED_EDGE('',*,*,#10138,.T.);
#14660=ORIENTED_EDGE('',*,*,#10081,.T.);
#14661=ORIENTED_EDGE('',*,*,#10080,.T.);
#14662=ORIENTED_EDGE('',*,*,#10079,.T.);
#14663=ORIENTED_EDGE('',*,*,#10139,.T.);
#14664=ORIENTED_EDGE('',*,*,#10073,.T.);
#14665=ORIENTED_EDGE('',*,*,#10140,.T.);
#14666=ORIENTED_EDGE('',*,*,#10074,.T.);
#14667=ORIENTED_EDGE('',*,*,#10139,.F.);
#14668=ORIENTED_EDGE('',*,*,#10078,.T.);
#14669=ORIENTED_EDGE('',*,*,#10077,.T.);
#14670=ORIENTED_EDGE('',*,*,#10076,.T.);
#14671=ORIENTED_EDGE('',*,*,#10141,.T.);
#14672=ORIENTED_EDGE('',*,*,#10142,.T.);
#14673=ORIENTED_EDGE('',*,*,#10143,.T.);
#14674=ORIENTED_EDGE('',*,*,#10088,.T.);
#14675=ORIENTED_EDGE('',*,*,#10087,.F.);
#14676=ORIENTED_EDGE('',*,*,#10086,.T.);
#14677=ORIENTED_EDGE('',*,*,#10085,.F.);
#14678=ORIENTED_EDGE('',*,*,#10144,.F.);
#14679=ORIENTED_EDGE('',*,*,#10145,.T.);
#14680=ORIENTED_EDGE('',*,*,#10091,.T.);
#14681=ORIENTED_EDGE('',*,*,#10090,.T.);
#14682=ORIENTED_EDGE('',*,*,#10089,.F.);
#14683=ORIENTED_EDGE('',*,*,#10143,.F.);
#14684=ORIENTED_EDGE('',*,*,#10146,.T.);
#14685=ORIENTED_EDGE('',*,*,#10147,.T.);
#14686=ORIENTED_EDGE('',*,*,#10071,.T.);
#14687=ORIENTED_EDGE('',*,*,#10148,.T.);
#14688=ORIENTED_EDGE('',*,*,#10149,.T.);
#14689=ORIENTED_EDGE('',*,*,#10150,.T.);
#14690=ORIENTED_EDGE('',*,*,#10151,.T.);
#14691=ORIENTED_EDGE('',*,*,#10152,.T.);
#14692=ORIENTED_EDGE('',*,*,#10153,.T.);
#14693=ORIENTED_EDGE('',*,*,#10154,.T.);
#14694=ORIENTED_EDGE('',*,*,#10155,.F.);
#14695=ORIENTED_EDGE('',*,*,#10098,.T.);
#14696=ORIENTED_EDGE('',*,*,#10097,.T.);
#14697=ORIENTED_EDGE('',*,*,#10096,.T.);
#14698=ORIENTED_EDGE('',*,*,#10156,.T.);
#14699=ORIENTED_EDGE('',*,*,#10155,.T.);
#14700=ORIENTED_EDGE('',*,*,#10156,.F.);
#14701=ORIENTED_EDGE('',*,*,#10095,.T.);
#14702=ORIENTED_EDGE('',*,*,#10094,.T.);
#14703=ORIENTED_EDGE('',*,*,#10093,.T.);
#14704=ORIENTED_EDGE('',*,*,#10157,.T.);
#14705=ORIENTED_EDGE('',*,*,#10084,.T.);
#14706=ORIENTED_EDGE('',*,*,#10157,.F.);
#14707=ORIENTED_EDGE('',*,*,#10092,.F.);
#14708=ORIENTED_EDGE('',*,*,#10145,.F.);
#14709=ORIENTED_EDGE('',*,*,#10144,.T.);
#14710=ORIENTED_EDGE('',*,*,#10075,.T.);
#14711=ORIENTED_EDGE('',*,*,#10124,.F.);
#14712=ORIENTED_EDGE('',*,*,#10082,.F.);
#14713=ORIENTED_EDGE('',*,*,#10141,.F.);
#14714=ORIENTED_EDGE('',*,*,#10149,.F.);
#14715=ORIENTED_EDGE('',*,*,#10154,.F.);
#14716=ORIENTED_EDGE('',*,*,#10153,.F.);
#14717=ORIENTED_EDGE('',*,*,#10152,.F.);
#14718=ORIENTED_EDGE('',*,*,#10158,.T.);
#14719=ORIENTED_EDGE('',*,*,#10142,.F.);
#14720=ORIENTED_EDGE('',*,*,#10146,.F.);
#14721=ORIENTED_EDGE('',*,*,#10158,.F.);
#14722=ORIENTED_EDGE('',*,*,#10151,.F.);
#14723=ORIENTED_EDGE('',*,*,#10150,.F.);
#14724=ORIENTED_EDGE('',*,*,#10070,.T.);
#14725=ORIENTED_EDGE('',*,*,#10140,.F.);
#14726=ORIENTED_EDGE('',*,*,#10072,.F.);
#14727=ORIENTED_EDGE('',*,*,#10147,.F.);
#14728=ORIENTED_EDGE('',*,*,#10148,.F.);
#14729=ORIENTED_EDGE('',*,*,#10138,.F.);
#14730=ORIENTED_EDGE('',*,*,#10159,.T.);
#14731=ORIENTED_EDGE('',*,*,#10135,.F.);
#14732=ORIENTED_EDGE('',*,*,#10159,.F.);
#14733=ORIENTED_EDGE('',*,*,#10137,.F.);
#14734=ORIENTED_EDGE('',*,*,#10160,.T.);
#14735=ORIENTED_EDGE('',*,*,#10133,.F.);
#14736=ORIENTED_EDGE('',*,*,#10160,.F.);
#14737=ORIENTED_EDGE('',*,*,#10110,.F.);
#14738=ORIENTED_EDGE('',*,*,#10161,.T.);
#14739=ORIENTED_EDGE('',*,*,#10108,.F.);
#14740=ORIENTED_EDGE('',*,*,#10161,.F.);
#16568=PLANE('',#18750);
#16569=PLANE('',#18762);
#16570=PLANE('',#18764);
#16571=PLANE('',#18785);
#16572=PLANE('',#18793);
#16573=PLANE('',#18800);
#16574=PLANE('',#18801);
#17253=ADVANCED_FACE('',(#4137),#1701,.T.);
#17254=ADVANCED_FACE('',(#4138),#1702,.F.);
#17255=ADVANCED_FACE('',(#4139),#1703,.T.);
#17256=ADVANCED_FACE('',(#4140,#3501),#16568,.F.);
#17257=ADVANCED_FACE('',(#4141),#3315,.T.);
#17258=ADVANCED_FACE('',(#4142),#16569,.T.);
#17259=ADVANCED_FACE('',(#4143,#3502),#16570,.T.);
#17260=ADVANCED_FACE('',(#4144),#3316,.F.);
#17261=ADVANCED_FACE('',(#4145,#3503),#3317,.F.);
#17262=ADVANCED_FACE('',(#4146),#3318,.F.);
#17263=ADVANCED_FACE('',(#4147),#3319,.F.);
#17264=ADVANCED_FACE('',(#4148),#3320,.T.);
#17265=ADVANCED_FACE('',(#4149),#3321,.T.);
#17266=ADVANCED_FACE('',(#4150),#3322,.T.);
#17267=ADVANCED_FACE('',(#4151),#3323,.T.);
#17268=ADVANCED_FACE('',(#4152),#3324,.T.);
#17269=ADVANCED_FACE('',(#4153,#3504),#16571,.T.);
#17270=ADVANCED_FACE('',(#4154),#235,.T.);
#17271=ADVANCED_FACE('',(#4155),#3325,.F.);
#17272=ADVANCED_FACE('',(#4156),#16572,.T.);
#17273=ADVANCED_FACE('',(#4157),#3326,.T.);
#17274=ADVANCED_FACE('',(#4158),#3327,.F.);
#17275=ADVANCED_FACE('',(#4159,#3505),#16573,.T.);
#17276=ADVANCED_FACE('',(#4160),#16574,.F.);
#17277=ADVANCED_FACE('',(#4161),#3328,.F.);
#17278=ADVANCED_FACE('',(#4162),#1704,.T.);
#17279=ADVANCED_FACE('',(#4163),#1705,.F.);
#17280=ADVANCED_FACE('',(#4164),#236,.T.);
#17281=ADVANCED_FACE('',(#4165),#1706,.T.);
#17282=ADVANCED_FACE('',(#4166),#237,.F.);
#17283=ADVANCED_FACE('',(#4167),#238,.T.);
#17284=ADVANCED_FACE('',(#4168),#239,.T.);
#17670=CLOSED_SHELL('',(#17253,#17254,#17255,#17256,#17257,#17258,#17259,
#17260,#17261,#17262,#17263,#17264,#17265,#17266,#17267,#17268,#17269,#17270,
#17271,#17272,#17273,#17274,#17275,#17276,#17277,#17278,#17279,#17280,#17281,
#17282,#17283,#17284));
#18747=AXIS2_PLACEMENT_3D('',#47199,#21697,#21698);
#18748=AXIS2_PLACEMENT_3D('',#47517,#21699,#21700);
#18749=AXIS2_PLACEMENT_3D('',#47623,#21701,#21702);
#18750=AXIS2_PLACEMENT_3D('',#47663,#21703,#21704);
#18751=AXIS2_PLACEMENT_3D('',#47665,#21705,#21706);
#18752=AXIS2_PLACEMENT_3D('',#47668,#21707,#21708);
#18753=AXIS2_PLACEMENT_3D('',#47670,#21709,#21710);
#18754=AXIS2_PLACEMENT_3D('',#47672,#21711,#21712);
#18755=AXIS2_PLACEMENT_3D('',#47674,#21713,#21714);
#18756=AXIS2_PLACEMENT_3D('',#47676,#21715,#21716);
#18757=AXIS2_PLACEMENT_3D('',#47678,#21717,#21718);
#18758=AXIS2_PLACEMENT_3D('',#47680,#21719,#21720);
#18759=AXIS2_PLACEMENT_3D('',#47681,#21721,#21722);
#18760=AXIS2_PLACEMENT_3D('',#47682,#21723,#21724);
#18761=AXIS2_PLACEMENT_3D('',#47684,#21725,#21726);
#18762=AXIS2_PLACEMENT_3D('',#47686,#21728,#21729);
#18763=AXIS2_PLACEMENT_3D('',#47688,#21730,#21731);
#18764=AXIS2_PLACEMENT_3D('',#47689,#21732,#21733);
#18765=AXIS2_PLACEMENT_3D('',#47692,#21734,#21735);
#18766=AXIS2_PLACEMENT_3D('',#47694,#21736,#21737);
#18767=AXIS2_PLACEMENT_3D('',#47696,#21738,#21739);
#18768=AXIS2_PLACEMENT_3D('',#47698,#21740,#21741);
#18769=AXIS2_PLACEMENT_3D('',#47700,#21742,#21743);
#18770=AXIS2_PLACEMENT_3D('',#47702,#21744,#21745);
#18771=AXIS2_PLACEMENT_3D('',#47704,#21746,#21747);
#18772=AXIS2_PLACEMENT_3D('',#47705,#21748,#21749);
#18773=AXIS2_PLACEMENT_3D('',#47707,#21750,#21751);
#18774=AXIS2_PLACEMENT_3D('',#47708,#21752,#21753);
#18775=AXIS2_PLACEMENT_3D('',#47711,#21756,#21757);
#18776=AXIS2_PLACEMENT_3D('',#47718,#21760,#21761);
#18777=AXIS2_PLACEMENT_3D('',#47721,#21764,#21765);
#18778=AXIS2_PLACEMENT_3D('',#47724,#21768,#21769);
#18779=AXIS2_PLACEMENT_3D('',#47725,#21770,#21771);
#18780=AXIS2_PLACEMENT_3D('',#47726,#21772,#21773);
#18781=AXIS2_PLACEMENT_3D('',#47727,#21774,#21775);
#18782=AXIS2_PLACEMENT_3D('',#47728,#21776,#21777);
#18783=AXIS2_PLACEMENT_3D('',#47732,#21779,#21780);
#18784=AXIS2_PLACEMENT_3D('',#47733,#21781,#21782);
#18785=AXIS2_PLACEMENT_3D('',#47734,#21783,#21784);
#18786=AXIS2_PLACEMENT_3D('',#47736,#21785,#21786);
#18787=AXIS2_PLACEMENT_3D('',#47738,#21787,#21788);
#18788=AXIS2_PLACEMENT_3D('',#47739,#21789,#21790);
#18789=AXIS2_PLACEMENT_3D('',#47740,#21791,#21792);
#18790=AXIS2_PLACEMENT_3D('',#47741,#21793,#21794);
#18791=AXIS2_PLACEMENT_3D('',#47743,#21795,#21796);
#18792=AXIS2_PLACEMENT_3D('',#47746,#21798,#21799);
#18793=AXIS2_PLACEMENT_3D('',#47747,#21800,#21801);
#18794=AXIS2_PLACEMENT_3D('',#47749,#21802,#21803);
#18795=AXIS2_PLACEMENT_3D('',#47750,#21804,#21805);
#18796=AXIS2_PLACEMENT_3D('',#47763,#21807,#21808);
#18797=AXIS2_PLACEMENT_3D('',#47766,#21809,#21810);
#18798=AXIS2_PLACEMENT_3D('',#47781,#21812,#21813);
#18799=AXIS2_PLACEMENT_3D('',#47782,#21814,#21815);
#18800=AXIS2_PLACEMENT_3D('',#47783,#21816,#21817);
#18801=AXIS2_PLACEMENT_3D('',#47868,#21818,#21819);
#18802=AXIS2_PLACEMENT_3D('',#47870,#21820,#21821);
#18803=AXIS2_PLACEMENT_3D('',#47871,#21822,#21823);
#18804=AXIS2_PLACEMENT_3D('',#47943,#21825,#21826);
#18805=AXIS2_PLACEMENT_3D('',#47944,#21827,#21828);
#18806=AXIS2_PLACEMENT_3D('',#47978,#21829,#21830);
#18807=AXIS2_PLACEMENT_3D('',#47979,#21831,#21832);
#18808=AXIS2_PLACEMENT_3D('',#47980,#21833,#21834);
#18809=AXIS2_PLACEMENT_3D('',#47981,#21835,#21836);
#18810=AXIS2_PLACEMENT_3D('',#47982,#21837,#21838);
#18811=AXIS2_PLACEMENT_3D('',#47983,#21839,#21840);
#21697=DIRECTION('axis',(0.,0.,1.));
#21698=DIRECTION('refdir',(1.,0.,0.));
#21699=DIRECTION('center_axis',(0.999262230046436,0.0296611786871826,-0.0243969277063748));
#21700=DIRECTION('ref_axis',(-0.00376824454709722,-0.556456744658462,-0.830868035043556));
#21701=DIRECTION('center_axis',(0.999262200442761,-0.0296605976385099,-0.0243988465714553));
#21702=DIRECTION('ref_axis',(0.00376825013598259,0.707931452975492,-0.706271093970949));
#21703=DIRECTION('center_axis',(-1.33376816360845E-16,1.,0.));
#21704=DIRECTION('ref_axis',(-1.,-1.33376816360845E-16,0.));
#21705=DIRECTION('center_axis',(-1.33376816360845E-16,1.,0.));
#21706=DIRECTION('ref_axis',(-1.,-1.33376816360845E-16,0.));
#21707=DIRECTION('center_axis',(-1.33376816360845E-16,1.,0.));
#21708=DIRECTION('ref_axis',(-1.,-1.33376816360845E-16,0.));
#21709=DIRECTION('center_axis',(-1.33376816360845E-16,1.,0.));
#21710=DIRECTION('ref_axis',(-1.,-1.33376816360845E-16,0.));
#21711=DIRECTION('center_axis',(-1.33376816360845E-16,1.,0.));
#21712=DIRECTION('ref_axis',(-1.,-1.33376816360845E-16,0.));
#21713=DIRECTION('center_axis',(-1.33376816360845E-16,1.,0.));
#21714=DIRECTION('ref_axis',(-1.,-1.33376816360845E-16,0.));
#21715=DIRECTION('center_axis',(-1.33376816360845E-16,1.,0.));
#21716=DIRECTION('ref_axis',(-1.,-1.33376816360845E-16,0.));
#21717=DIRECTION('center_axis',(-1.33376816360845E-16,1.,0.));
#21718=DIRECTION('ref_axis',(-1.,-1.33376816360845E-16,0.));
#21719=DIRECTION('center_axis',(-1.33376816360845E-16,1.,0.));
#21720=DIRECTION('ref_axis',(-1.,-1.33376816360845E-16,0.));
#21721=DIRECTION('center_axis',(-1.33376816360845E-16,1.,0.));
#21722=DIRECTION('ref_axis',(-1.,-1.33376816360845E-16,0.));
#21723=DIRECTION('center_axis',(-1.33376816360845E-16,1.,0.));
#21724=DIRECTION('ref_axis',(-1.,-1.33376816360845E-16,0.));
#21725=DIRECTION('center_axis',(-1.33376816360845E-16,1.,0.));
#21726=DIRECTION('ref_axis',(-1.,-1.33376816360845E-16,0.));
#21727=DIRECTION('',(1.33376816360845E-16,-1.,0.));
#21728=DIRECTION('center_axis',(-1.33376816360845E-16,1.,0.));
#21729=DIRECTION('ref_axis',(-1.,-1.33376816360845E-16,0.));
#21730=DIRECTION('center_axis',(-1.33376816360845E-16,1.,0.));
#21731=DIRECTION('ref_axis',(-1.,-1.33376816360845E-16,0.));
#21732=DIRECTION('center_axis',(1.15648231731787E-16,-1.,0.));
#21733=DIRECTION('ref_axis',(1.,1.15648231731787E-16,0.));
#21734=DIRECTION('center_axis',(1.15648231731787E-16,-1.,0.));
#21735=DIRECTION('ref_axis',(1.,1.15648231731787E-16,0.));
#21736=DIRECTION('center_axis',(1.15648231731787E-16,-1.,0.));
#21737=DIRECTION('ref_axis',(1.,1.15648231731787E-16,0.));
#21738=DIRECTION('center_axis',(1.15648231731787E-16,-1.,0.));
#21739=DIRECTION('ref_axis',(1.,1.15648231731787E-16,0.));
#21740=DIRECTION('center_axis',(1.15648231731787E-16,-1.,0.));
#21741=DIRECTION('ref_axis',(1.,1.15648231731787E-16,0.));
#21742=DIRECTION('center_axis',(1.15648231731787E-16,-1.,0.));
#21743=DIRECTION('ref_axis',(1.,1.15648231731787E-16,0.));
#21744=DIRECTION('center_axis',(1.15648231731787E-16,-1.,0.));
#21745=DIRECTION('ref_axis',(1.,1.15648231731787E-16,0.));
#21746=DIRECTION('center_axis',(1.15648231731787E-16,-1.,0.));
#21747=DIRECTION('ref_axis',(1.,1.15648231731787E-16,0.));
#21748=DIRECTION('center_axis',(1.15648231731787E-16,-1.,0.));
#21749=DIRECTION('ref_axis',(1.,1.15648231731787E-16,0.));
#21750=DIRECTION('center_axis',(1.15648231731787E-16,-1.,0.));
#21751=DIRECTION('ref_axis',(1.,1.15648231731787E-16,0.));
#21752=DIRECTION('center_axis',(-9.13012355777267E-17,1.,0.));
#21753=DIRECTION('ref_axis',(-1.,-9.13012355777267E-17,0.));
#21754=DIRECTION('',(-9.13012355777267E-17,1.,0.));
#21755=DIRECTION('',(-9.13012355777267E-17,1.,0.));
#21756=DIRECTION('center_axis',(-1.33376816360844E-16,1.,4.20755807831181E-17));
#21757=DIRECTION('ref_axis',(1.,1.33376816360845E-16,-1.2312033195887E-14));
#21758=DIRECTION('',(-1.33376816360844E-16,1.,4.20755807831181E-17));
#21759=DIRECTION('',(-1.33376816360844E-16,1.,4.20755807831181E-17));
#21760=DIRECTION('center_axis',(-1.33376816360845E-16,1.,-4.20755807831181E-17));
#21761=DIRECTION('ref_axis',(-1.,-1.33376816360845E-16,0.));
#21762=DIRECTION('',(-1.33376816360845E-16,1.,-4.20755807831181E-17));
#21763=DIRECTION('',(-1.33376816360845E-16,1.,-4.20755807831181E-17));
#21764=DIRECTION('center_axis',(-1.75452397143963E-16,1.,0.));
#21765=DIRECTION('ref_axis',(-1.,-1.75452397143963E-16,0.));
#21766=DIRECTION('',(-1.75452397143963E-16,1.,0.));
#21767=DIRECTION('',(-1.75452397143963E-16,1.,0.));
#21768=DIRECTION('center_axis',(-1.75452397143963E-16,1.,0.));
#21769=DIRECTION('ref_axis',(-1.,-1.75452397143963E-16,0.));
#21770=DIRECTION('center_axis',(-1.33376816360845E-16,1.,-4.20755807831181E-17));
#21771=DIRECTION('ref_axis',(0.707106781186543,6.45597228077203E-17,-0.707106781186552));
#21772=DIRECTION('center_axis',(-9.13012355777267E-17,1.,0.));
#21773=DIRECTION('ref_axis',(0.707106781186543,6.45597228077206E-17,0.707106781186552));
#21774=DIRECTION('center_axis',(-1.33376816360844E-16,1.,4.20755807831181E-17));
#21775=DIRECTION('ref_axis',(-1.,-1.33376816360844E-16,0.));
#21776=DIRECTION('center_axis',(-1.15648231731787E-16,1.,0.));
#21777=DIRECTION('ref_axis',(-1.,-1.15648231731787E-16,0.));
#21778=DIRECTION('',(1.15648231731787E-16,-1.,0.));
#21779=DIRECTION('center_axis',(1.15648231731787E-16,-1.,0.));
#21780=DIRECTION('ref_axis',(1.,1.15648231731787E-16,0.));
#21781=DIRECTION('center_axis',(1.15648231731787E-16,-1.,0.));
#21782=DIRECTION('ref_axis',(1.,1.15648231731787E-16,0.));
#21783=DIRECTION('center_axis',(1.15648231731787E-16,-1.,0.));
#21784=DIRECTION('ref_axis',(1.,1.15648231731787E-16,0.));
#21785=DIRECTION('center_axis',(1.15648231731787E-16,-1.,0.));
#21786=DIRECTION('ref_axis',(1.,1.15648231731787E-16,0.));
#21787=DIRECTION('center_axis',(1.15648231731787E-16,-1.,0.));
#21788=DIRECTION('ref_axis',(1.,1.15648231731787E-16,0.));
#21789=DIRECTION('center_axis',(1.15648231731787E-16,-1.,0.));
#21790=DIRECTION('ref_axis',(1.,0.,0.));
#21791=DIRECTION('center_axis',(1.22464679914735E-16,1.41628236817384E-32,
-1.));
#21792=DIRECTION('ref_axis',(-1.,0.,-1.22464679914735E-16));
#21793=DIRECTION('center_axis',(1.15648231731787E-16,-1.,0.));
#21794=DIRECTION('ref_axis',(1.,1.15648231731787E-16,0.));
#21795=DIRECTION('center_axis',(1.15648231731787E-16,-1.,0.));
#21796=DIRECTION('ref_axis',(1.,1.15648231731787E-16,0.));
#21797=DIRECTION('',(1.15648231731787E-16,-1.,0.));
#21798=DIRECTION('center_axis',(1.15648231731787E-16,-1.,0.));
#21799=DIRECTION('ref_axis',(1.,1.15648231731787E-16,0.));
#21800=DIRECTION('center_axis',(1.15648231731787E-16,-1.,0.));
#21801=DIRECTION('ref_axis',(1.,1.15648231731787E-16,0.));
#21802=DIRECTION('center_axis',(1.15648231731787E-16,-1.,0.));
#21803=DIRECTION('ref_axis',(1.,1.15648231731787E-16,0.));
#21804=DIRECTION('center_axis',(1.,4.38931774757775E-24,-9.9579925010296E-17));
#21805=DIRECTION('ref_axis',(-9.9579925010296E-17,0.,-1.));
#21806=DIRECTION('',(-1.,-4.38931774757775E-24,9.9579925010296E-17));
#21807=DIRECTION('center_axis',(1.,-2.11863444194148E-23,-9.9579925010296E-17));
#21808=DIRECTION('ref_axis',(-9.9579925010296E-17,0.,-1.));
#21809=DIRECTION('center_axis',(-1.,1.98089019303025E-8,-1.56581200582727E-8));
#21810=DIRECTION('ref_axis',(2.43121132745886E-8,0.587909515445564,-0.80892669732712));
#21811=DIRECTION('',(1.,-2.11863444194148E-23,-9.9579925010296E-17));
#21812=DIRECTION('center_axis',(0.999472141255957,-0.0286348071154382,-0.0153455750851244));
#21813=DIRECTION('ref_axis',(0.00317408767800045,0.556162888203051,-0.831067245746729));
#21814=DIRECTION('center_axis',(-1.,1.98089019303025E-8,-1.56581200582727E-8));
#21815=DIRECTION('ref_axis',(2.43121132745886E-8,0.587909515445564,-0.80892669732712));
#21816=DIRECTION('center_axis',(-1.,0.,0.));
#21817=DIRECTION('ref_axis',(0.,0.,1.));
#21818=DIRECTION('center_axis',(1.,0.,0.));
#21819=DIRECTION('ref_axis',(0.,0.,-1.));
#21820=DIRECTION('center_axis',(1.,0.,0.));
#21821=DIRECTION('ref_axis',(0.,0.,-1.));
#21822=DIRECTION('center_axis',(1.,0.,0.));
#21823=DIRECTION('ref_axis',(0.,0.,-1.));
#21824=DIRECTION('',(1.,0.,0.));
#21825=DIRECTION('center_axis',(0.999999999993368,5.57549682629954E-7,-3.59912391188234E-6));
#21826=DIRECTION('ref_axis',(-3.59912391187535E-6,0.,-0.999999999993523));
#21827=DIRECTION('center_axis',(5.57549682626343E-7,-0.999999999999845,
-2.00669039482449E-12));
#21828=DIRECTION('ref_axis',(3.59912391189779E-6,0.,0.999999999993523));
#21829=DIRECTION('center_axis',(1.15648231731787E-16,-1.,0.));
#21830=DIRECTION('ref_axis',(1.,0.,0.));
#21831=DIRECTION('center_axis',(-1.22464679914735E-16,-1.41628236817384E-32,
1.));
#21832=DIRECTION('ref_axis',(-1.,0.,-1.22464679914735E-16));
#21833=DIRECTION('center_axis',(1.15648231731787E-16,-1.,0.));
#21834=DIRECTION('ref_axis',(1.,0.,0.));
#21835=DIRECTION('center_axis',(1.22464679914735E-16,1.41628236817384E-32,
-1.));
#21836=DIRECTION('ref_axis',(-1.,0.,-1.22464679914735E-16));
#21837=DIRECTION('center_axis',(-1.33376816360845E-16,1.,0.));
#21838=DIRECTION('ref_axis',(-1.,0.,0.));
#21839=DIRECTION('center_axis',(-1.22464679914735E-16,-1.63339491236773E-32,
-1.));
#21840=DIRECTION('ref_axis',(1.,0.,-1.22464679914735E-16));
#47199=CARTESIAN_POINT('',(0.,0.,0.));
#47200=CARTESIAN_POINT('Ctrl Pts',(-0.00380975858063242,-0.00881478413029403,
-0.00183246684420301));
#47201=CARTESIAN_POINT('Ctrl Pts',(-0.00390993294014545,-0.00881478413029403,
-0.00183246684420301));
#47202=CARTESIAN_POINT('Ctrl Pts',(-0.00390975842889103,-0.00882512165273333,
-0.00173282745701358));
#47203=CARTESIAN_POINT('Ctrl Pts',(-0.00380975858063242,-0.00929465142715738,
-0.0018806998537358));
#47204=CARTESIAN_POINT('Ctrl Pts',(-0.00390993294014545,-0.00929465142715738,
-0.0018806998537358));
#47205=CARTESIAN_POINT('Ctrl Pts',(-0.00390975842889103,-0.00927906675289324,
-0.00177836203380147));
#47206=CARTESIAN_POINT('Ctrl Pts',(-0.00380975858063242,-0.0102936387094841,
-0.00158253456509613));
#47207=CARTESIAN_POINT('Ctrl Pts',(-0.00390993294014546,-0.0102936387094841,
-0.00158253456509614));
#47208=CARTESIAN_POINT('Ctrl Pts',(-0.00390975842889104,-0.0102241270617854,
-0.00149607241763065));
#47209=CARTESIAN_POINT('Ctrl Pts',(-0.00380975858063242,-0.0110403459009329,
-0.000207601983482724));
#47210=CARTESIAN_POINT('Ctrl Pts',(-0.00390993294014544,-0.0110403459009329,
-0.000207601983482722));
#47211=CARTESIAN_POINT('Ctrl Pts',(-0.00390975842889102,-0.0109298209858678,
-0.00019577210929604));
#47212=CARTESIAN_POINT('Ctrl Pts',(-0.00380975858063243,-0.010585488822892,
0.00129440175744357));
#47213=CARTESIAN_POINT('Ctrl Pts',(-0.00390993294014546,-0.010585488822892,
0.00129440175744357));
#47214=CARTESIAN_POINT('Ctrl Pts',(-0.00390975842889104,-0.0104994209642949,
0.0012241417666484));
#47215=CARTESIAN_POINT('Ctrl Pts',(-0.00380975858063242,-0.00920314460986179,
0.00202990873817867));
#47216=CARTESIAN_POINT('Ctrl Pts',(-0.00390993294014544,-0.00920314460986179,
0.00202990873817867));
#47217=CARTESIAN_POINT('Ctrl Pts',(-0.00390975842889102,-0.00919187984963056,
0.00191958960744435));
#47218=CARTESIAN_POINT('Ctrl Pts',(-0.00380975858063242,-0.00770446035061261,
0.0015817160659287));
#47219=CARTESIAN_POINT('Ctrl Pts',(-0.00390993294014545,-0.00770446035061261,
0.0015817160659287));
#47220=CARTESIAN_POINT('Ctrl Pts',(-0.00390975842889103,-0.00777409310458325,
0.00149536140507255));
#47221=CARTESIAN_POINT('Ctrl Pts',(-0.00380975858063242,-0.00695993177951074,
0.000203870131802003));
#47222=CARTESIAN_POINT('Ctrl Pts',(-0.00390993294014545,-0.00695993177951073,
0.000203870131802006));
#47223=CARTESIAN_POINT('Ctrl Pts',(-0.00390975842889103,-0.00707045087524681,
0.000192132115288156));
#47224=CARTESIAN_POINT('Ctrl Pts',(-0.00380975858063242,-0.00741443492830406,
-0.00129313650789938));
#47225=CARTESIAN_POINT('Ctrl Pts',(-0.00390993294014545,-0.00741443492830407,
-0.00129313650789939));
#47226=CARTESIAN_POINT('Ctrl Pts',(-0.00390975842889103,-0.00750045646082591,
-0.00122286495690331));
#47227=CARTESIAN_POINT('Ctrl Pts',(-0.00380975858063242,-0.00833491683343068,
-0.00178423383467021));
#47228=CARTESIAN_POINT('Ctrl Pts',(-0.00390993294014545,-0.00833491683343068,
-0.00178423383467021));
#47229=CARTESIAN_POINT('Ctrl Pts',(-0.00390975842889103,-0.00837117655257341,
-0.00168729288022569));
#47230=CARTESIAN_POINT('Ctrl Pts',(-0.00380975858063242,-0.00881478413029403,
-0.00183246684420301));
#47231=CARTESIAN_POINT('Ctrl Pts',(-0.00390993294014545,-0.00881478413029403,
-0.00183246684420301));
#47232=CARTESIAN_POINT('Ctrl Pts',(-0.00390975842889103,-0.00882512165273333,
-0.00173282745701358));
#47233=CARTESIAN_POINT('',(-0.00390975858063242,-0.00882510339125232,-0.00173300347273605));
#47234=CARTESIAN_POINT('',(-0.00380975858063243,-0.00881478413029403,-0.00183246684420301));
#47235=CARTESIAN_POINT('Ctrl Pts',(-0.00390975857180975,-0.00882509934044699,
-0.00173304251652624));
#47236=CARTESIAN_POINT('Ctrl Pts',(-0.0039097165831011,-0.00881478413029403,
-0.00183246684420301));
#47237=CARTESIAN_POINT('Ctrl Pts',(-0.00380975858063242,-0.00881478413029403,
-0.00183246684420301));
#47238=CARTESIAN_POINT('',(-0.00390975858063242,-0.00900031988990579,-0.00174210523730213));
#47239=CARTESIAN_POINT('Ctrl Pts',(-0.00390975858063242,-0.0090003198899058,
-0.00174210523730213));
#47240=CARTESIAN_POINT('Ctrl Pts',(-0.00390975858063242,-0.00945687992322838,
-0.00174202447630927));
#47241=CARTESIAN_POINT('Ctrl Pts',(-0.00390975858063242,-0.0103697614232141,
-0.00136637602002286));
#47242=CARTESIAN_POINT('Ctrl Pts',(-0.00390975858063242,-0.0109405594065751,
-2.90486592512132E-7));
#47243=CARTESIAN_POINT('Ctrl Pts',(-0.00390975858063242,-0.0103680426596137,
0.00136935520820644));
#47244=CARTESIAN_POINT('Ctrl Pts',(-0.00390975858063243,-0.00899628845176151,
0.00192951445904318));
#47245=CARTESIAN_POINT('Ctrl Pts',(-0.00390975858063241,-0.00762974915067706,
0.00136520476073566));
#47246=CARTESIAN_POINT('Ctrl Pts',(-0.00390975858063243,-0.00706013247825494,
8.11459216446678E-7));
#47247=CARTESIAN_POINT('Ctrl Pts',(-0.00390975858063242,-0.00760544730692673,
-0.00130817127168898));
#47248=CARTESIAN_POINT('Ctrl Pts',(-0.00390975858063242,-0.00842870221548062,
-0.00169187672673672));
#47249=CARTESIAN_POINT('Ctrl Pts',(-0.00390975858063242,-0.00882510339125232,
-0.00173300347273605));
#47250=CARTESIAN_POINT('',(-0.00380975858063243,-0.00899998937218426,-0.00184137848958098));
#47251=CARTESIAN_POINT('Ctrl Pts',(-0.00390975606002064,-0.00900031988985028,
-0.00174210521939449));
#47252=CARTESIAN_POINT('Ctrl Pts',(-0.00390905107214187,-0.00899998937218426,
-0.00184137848958098));
#47253=CARTESIAN_POINT('Ctrl Pts',(-0.00380975858063242,-0.00899998937218426,
-0.00184137848958098));
#47254=CARTESIAN_POINT('',(-0.00380975858063243,-0.00900001212691424,0.00184141020097112));
#47255=CARTESIAN_POINT('Ctrl Pts',(-0.00380975858063243,-0.00900001212691424,
0.00184141020097112));
#47256=CARTESIAN_POINT('Ctrl Pts',(-0.00380975858063243,-0.00906142348782768,
0.00184161153465334));
#47257=CARTESIAN_POINT('Ctrl Pts',(-0.00380975858063243,-0.00912270322366649,
0.00183871389074159));
#47258=CARTESIAN_POINT('Ctrl Pts',(-0.00380975858063243,-0.00918375460215863,
0.00183262546268116));
#47259=CARTESIAN_POINT('Ctrl Pts',(-0.00380975858063243,-0.00966332758164447,
0.00178479942406512));
#47260=CARTESIAN_POINT('Ctrl Pts',(-0.00380975858063243,-0.0101244136873442,
0.00153992848358091));
#47261=CARTESIAN_POINT('Ctrl Pts',(-0.00380975858063243,-0.0104309076337271,
0.0011666522974117));
#47262=CARTESIAN_POINT('Ctrl Pts',(-0.00380975858063243,-0.0107366396990011,
0.000794303999306896));
#47263=CARTESIAN_POINT('Ctrl Pts',(-0.00380975858063243,-0.0108887999330076,
0.000293786106230727));
#47264=CARTESIAN_POINT('Ctrl Pts',(-0.00380975858063243,-0.0108400851893513,
-0.000186423456930577));
#47265=CARTESIAN_POINT('Ctrl Pts',(-0.00380975858063243,-0.0107914327883849,
-0.000666018471935143));
#47266=CARTESIAN_POINT('Ctrl Pts',(-0.00380975858063243,-0.0105418163288552,
-0.00112481192963245));
#47267=CARTESIAN_POINT('Ctrl Pts',(-0.00380975858063243,-0.0101683430874772,
-0.00142792045698715));
#47268=CARTESIAN_POINT('Ctrl Pts',(-0.00380975858063243,-0.00984183803121622,
-0.00169290990151061));
#47269=CARTESIAN_POINT('Ctrl Pts',(-0.00380975858063243,-0.00941977782130047,
-0.00183994022345956));
#47270=CARTESIAN_POINT('Ctrl Pts',(-0.00380975858063243,-0.00899998937218426,
-0.00184137848958098));
#47271=CARTESIAN_POINT('Ctrl Pts',(-0.00380975858063243,-0.00881478413029403,
-0.00183246684420301));
#47272=CARTESIAN_POINT('Ctrl Pts',(-0.00380975858063243,-0.00833564521297648,
-0.00178430704644731));
#47273=CARTESIAN_POINT('Ctrl Pts',(-0.00380975858063243,-0.00787521215159384,
-0.00153933786611053));
#47274=CARTESIAN_POINT('Ctrl Pts',(-0.00380975858063243,-0.00756880487978684,
-0.0011664097329752));
#47275=CARTESIAN_POINT('Ctrl Pts',(-0.00380975858063243,-0.00726345873171947,
-0.000794773092998356));
#47276=CARTESIAN_POINT('Ctrl Pts',(-0.00380975858063243,-0.00711142381370158,
-0.000295221445893798));
#47277=CARTESIAN_POINT('Ctrl Pts',(-0.00380975858063243,-0.00715977039949327,
0.000184010014206217));
#47278=CARTESIAN_POINT('Ctrl Pts',(-0.00380975858063243,-0.00720817502841981,
0.000663816821992245));
#47279=CARTESIAN_POINT('Ctrl Pts',(-0.00380975858063243,-0.00745702122447455,
0.0011230340789884));
#47280=CARTESIAN_POINT('Ctrl Pts',(-0.00380975858063243,-0.00783015296530383,
0.00142677385561591));
#47281=CARTESIAN_POINT('Ctrl Pts',(-0.00380975858063243,-0.00815677065544411,
0.00169264988113258));
#47282=CARTESIAN_POINT('Ctrl Pts',(-0.00380975858063243,-0.00857913028022675,
0.00184003036358083));
#47283=CARTESIAN_POINT('Ctrl Pts',(-0.00380975858063243,-0.00900001212691424,
0.00184141020097112));
#47284=CARTESIAN_POINT('Ctrl Pts',(-0.0035392791351489,-0.00858849912814965,
-0.00179466521288696));
#47285=CARTESIAN_POINT('Ctrl Pts',(-0.00342573153923465,-0.00859176400850957,
-0.00179333404984997));
#47286=CARTESIAN_POINT('Ctrl Pts',(-0.00343811948343117,-0.00856602524158671,
-0.00190328650635992));
#47287=CARTESIAN_POINT('Ctrl Pts',(-0.00355142559943888,-0.00905859136078448,
-0.00190144952999438));
#47288=CARTESIAN_POINT('Ctrl Pts',(-0.00343722171108695,-0.00906840205799737,
-0.00190374929419889));
#47289=CARTESIAN_POINT('Ctrl Pts',(-0.0034503400565124,-0.00906157284819796,
-0.0020166590821151));
#47290=CARTESIAN_POINT('Ctrl Pts',(-0.00352537010396588,-0.0100884377158575,
-0.00172789987787408));
#47291=CARTESIAN_POINT('Ctrl Pts',(-0.0034151603753512,-0.0100497091309754,
-0.00174559426658833));
#47292=CARTESIAN_POINT('Ctrl Pts',(-0.00342416641781692,-0.0101460057925454,
-0.00183316467220812));
#47293=CARTESIAN_POINT('Ctrl Pts',(-0.00341335748290235,-0.0109970962519671,
-0.000457281663563109));
#47294=CARTESIAN_POINT('Ctrl Pts',(-0.00331425963473675,-0.010996887331939,
-0.000476856829642387));
#47295=CARTESIAN_POINT('Ctrl Pts',(-0.0033115684832145,-0.0111050748119872,
-0.000486036946141634));
#47296=CARTESIAN_POINT('Ctrl Pts',(-0.00345233946123927,-0.0107338060170907,
0.00108652455487473));
#47297=CARTESIAN_POINT('Ctrl Pts',(-0.00335032457735252,-0.0107129565277369,
0.00112100474052161));
#47298=CARTESIAN_POINT('Ctrl Pts',(-0.00335076613415529,-0.0108274712600009,
0.00115282043607336));
#47299=CARTESIAN_POINT('Ctrl Pts',(-0.00356449374860163,-0.00945621932640169,
0.00198829625682747));
#47300=CARTESIAN_POINT('Ctrl Pts',(-0.00344854884364189,-0.00943365667565594,
0.00198475236629158));
#47301=CARTESIAN_POINT('Ctrl Pts',(-0.0034634722557383,-0.00948068538942303,
0.00210854197031486));
#47302=CARTESIAN_POINT('Ctrl Pts',(-0.00352531374816938,-0.00791032423527775,
0.00172792526671951));
#47303=CARTESIAN_POINT('Ctrl Pts',(-0.00341511348123987,-0.00794907951679388,
0.00174568140804206));
#47304=CARTESIAN_POINT('Ctrl Pts',(-0.00342410980697788,-0.0078526998577211,
0.00183315731298699));
#47305=CARTESIAN_POINT('Ctrl Pts',(-0.00341328178572483,-0.00700287546046352,
0.000454633913679566));
#47306=CARTESIAN_POINT('Ctrl Pts',(-0.00331419107940177,-0.00700305969526376,
0.000474177195847323));
#47307=CARTESIAN_POINT('Ctrl Pts',(-0.00331149240063511,-0.00689487285927746,
0.000483300740605997));
#47308=CARTESIAN_POINT('Ctrl Pts',(-0.00345241595160808,-0.00726632486312327,
-0.00108656836792835));
#47309=CARTESIAN_POINT('Ctrl Pts',(-0.00335038976344317,-0.00728717254733531,
-0.00112102914438496));
#47310=CARTESIAN_POINT('Ctrl Pts',(-0.00335084297932956,-0.00717272015287796,
-0.00115292921767708));
#47311=CARTESIAN_POINT('Ctrl Pts',(-0.00352712997637068,-0.00811830261348138,
-0.00168785720747976));
#47312=CARTESIAN_POINT('Ctrl Pts',(-0.00341440081056064,-0.00812174001897434,
-0.00168445098079964));
#47313=CARTESIAN_POINT('Ctrl Pts',(-0.00342589891034995,-0.00807047763497546,
-0.00178991393060475));
#47314=CARTESIAN_POINT('Ctrl Pts',(-0.0035392791351489,-0.00858849912814965,
-0.00179466521288696));
#47315=CARTESIAN_POINT('Ctrl Pts',(-0.00342573153923465,-0.00859176400850957,
-0.00179333404984997));
#47316=CARTESIAN_POINT('Ctrl Pts',(-0.00343811948343117,-0.00856602524158671,
-0.00190328650635992));
#47317=CARTESIAN_POINT('',(-0.00353642309488705,-0.00858783002638803,-0.00179790810359568));
#47318=CARTESIAN_POINT('',(-0.00343811948343117,-0.00856602524158671,-0.00190328650635992));
#47319=CARTESIAN_POINT('Ctrl Pts',(-0.00353638626969755,-0.00858857287636746,
-0.0017946721002847));
#47320=CARTESIAN_POINT('Ctrl Pts',(-0.00342608713477122,-0.00859102517803947,
-0.00179649023154958));
#47321=CARTESIAN_POINT('Ctrl Pts',(-0.00343811948343117,-0.00856602524158671,
-0.00190328650635992));
#47322=CARTESIAN_POINT('',(-0.00346348111810162,-0.00743152690402934,-0.000970909650152327));
#47323=CARTESIAN_POINT('Ctrl Pts',(-0.00346348111810161,-0.00743152690402934,
-0.000970909650152327));
#47324=CARTESIAN_POINT('Ctrl Pts',(-0.00346891490008736,-0.00748743871269397,
-0.00106078753922695));
#47325=CARTESIAN_POINT('Ctrl Pts',(-0.00347494633059866,-0.00755249303664913,
-0.0011489837185329));
#47326=CARTESIAN_POINT('Ctrl Pts',(-0.00348147326192271,-0.00762799489769548,
-0.00123298157944914));
#47327=CARTESIAN_POINT('Ctrl Pts',(-0.00349040136462214,-0.00773127289097472,
-0.00134788113814814));
#47328=CARTESIAN_POINT('Ctrl Pts',(-0.00350025660587228,-0.00785531577230295,
-0.00145410062115423));
#47329=CARTESIAN_POINT('Ctrl Pts',(-0.00350830630757828,-0.00797937744348274,
-0.00153649554303844));
#47330=CARTESIAN_POINT('Ctrl Pts',(-0.00351635600928428,-0.00810343911466254,
-0.00161889046492264));
#47331=CARTESIAN_POINT('Ctrl Pts',(-0.00352260017144614,-0.00822631358203606,
-0.00167942932986295));
#47332=CARTESIAN_POINT('Ctrl Pts',(-0.00352769155837584,-0.0083470181408938,
-0.00172511126229019));
#47333=CARTESIAN_POINT('Ctrl Pts',(-0.00353115476696423,-0.00842912250079946,
-0.00175618453621361));
#47334=CARTESIAN_POINT('Ctrl Pts',(-0.00353408460414614,-0.00851028574239199,
-0.0017800585327765));
#47335=CARTESIAN_POINT('Ctrl Pts',(-0.00353642309488705,-0.00858783002638803,
-0.00179790810359568));
#47336=CARTESIAN_POINT('',(-0.00351047268888782,-0.00801620582113018,0.00156083213605469));
#47337=CARTESIAN_POINT('Ctrl Pts',(-0.00351047268888782,-0.00801620582113018,
0.00156083213605469));
#47338=CARTESIAN_POINT('Ctrl Pts',(-0.00350519018615136,-0.00792957352973586,
0.0015060133715871));
#47339=CARTESIAN_POINT('Ctrl Pts',(-0.0034993421679523,-0.00784462670554804,
0.00144258322748745));
#47340=CARTESIAN_POINT('Ctrl Pts',(-0.00349300905755829,-0.00776351543005723,
0.00136932733695487));
#47341=CARTESIAN_POINT('Ctrl Pts',(-0.00348450377901836,-0.00765458412334417,
0.00127094570219624));
#47342=CARTESIAN_POINT('Ctrl Pts',(-0.00347512358267887,-0.00755333188928983,
0.0011538009990632));
#47343=CARTESIAN_POINT('Ctrl Pts',(-0.00346735993405672,-0.00747341176998912,
0.00103600768938707));
#47344=CARTESIAN_POINT('Ctrl Pts',(-0.00345959628543458,-0.00739349165068841,
0.000918214379710948));
#47345=CARTESIAN_POINT('Ctrl Pts',(-0.0034534491845298,-0.00733336819546107,
0.000800677106835236));
#47346=CARTESIAN_POINT('Ctrl Pts',(-0.00344838046399713,-0.00728767396264777,
0.000686692944772953));
#47347=CARTESIAN_POINT('Ctrl Pts',(-0.00343824302293181,-0.00719628549702117,
0.00045872462064838));
#47348=CARTESIAN_POINT('Ctrl Pts',(-0.00343241910335498,-0.00716194741939409,
0.00024557134629273));
#47349=CARTESIAN_POINT('Ctrl Pts',(-0.00343139975819657,-0.00715609923797259,
5.76277457690076E-5));
#47350=CARTESIAN_POINT('Ctrl Pts',(-0.0034308900856098,-0.00715317514721843,
-3.63440558877464E-5));
#47351=CARTESIAN_POINT('Ctrl Pts',(-0.00343158155666329,-0.00715675113122004,
-0.000123973903842955));
#47352=CARTESIAN_POINT('Ctrl Pts',(-0.0034334038173975,-0.00716863494412438,
-0.000221928606050654));
#47353=CARTESIAN_POINT('Ctrl Pts',(-0.00343522607813171,-0.00718051875702871,
-0.000319883308258354));
#47354=CARTESIAN_POINT('Ctrl Pts',(-0.00343817912854665,-0.00720169129494195,
-0.000428004954841905));
#47355=CARTESIAN_POINT('Ctrl Pts',(-0.00344241723298215,-0.0072364971068012,
-0.000541338231156834));
#47356=CARTESIAN_POINT('Ctrl Pts',(-0.00344763208804926,-0.00727932457061238,
-0.00068079128599747));
#47357=CARTESIAN_POINT('Ctrl Pts',(-0.00345479258345437,-0.00734336632775489,
-0.000827815016986945));
#47358=CARTESIAN_POINT('Ctrl Pts',(-0.00346348111810161,-0.00743152690402934,
-0.000970909650152327));
#47359=CARTESIAN_POINT('',(-0.00354320482548136,-0.00900000021011351,0.00184504509674603));
#47360=CARTESIAN_POINT('Ctrl Pts',(-0.00354320482548136,-0.00900000021011351,
0.00184504509674603));
#47361=CARTESIAN_POINT('Ctrl Pts',(-0.00354322509066825,-0.00892539297133586,
0.00184524864599605));
#47362=CARTESIAN_POINT('Ctrl Pts',(-0.00354247918437561,-0.00885283033216195,
0.00184089127245303));
#47363=CARTESIAN_POINT('Ctrl Pts',(-0.00354100586630036,-0.00877374298082574,
0.00183111770926393));
#47364=CARTESIAN_POINT('Ctrl Pts',(-0.0035391715477079,-0.00867527721065587,
0.00181894937374049));
#47365=CARTESIAN_POINT('Ctrl Pts',(-0.00353620967645606,-0.00856685861537494,
0.00179739568288771));
#47366=CARTESIAN_POINT('Ctrl Pts',(-0.00353198328180325,-0.00845354303295786,
0.00176225261832798));
#47367=CARTESIAN_POINT('Ctrl Pts',(-0.00352667750664014,-0.00831128774158746,
0.0017181343533731));
#47368=CARTESIAN_POINT('Ctrl Pts',(-0.00351937883628627,-0.00816158475318592,
0.0016521136331202));
#47369=CARTESIAN_POINT('Ctrl Pts',(-0.00351047268888782,-0.00801620582113018,
0.00156083213605469));
#47370=CARTESIAN_POINT('',(-0.0034634765427239,-0.0105683977214321,0.000971535379578606));
#47371=CARTESIAN_POINT('Ctrl Pts',(-0.0034634765427239,-0.0105683977214321,
0.000971535379578606));
#47372=CARTESIAN_POINT('Ctrl Pts',(-0.00346890409325003,-0.0105125988361509,
0.00106128251009728));
#47373=CARTESIAN_POINT('Ctrl Pts',(-0.00347493845705885,-0.010447588087778,
0.00114939417218175));
#47374=CARTESIAN_POINT('Ctrl Pts',(-0.00348148957894286,-0.0103720280455907,
0.0012334598492987));
#47375=CARTESIAN_POINT('Ctrl Pts',(-0.00349000372301041,-0.0102738266846141,
0.00134271553081146));
#47376=CARTESIAN_POINT('Ctrl Pts',(-0.00349939071363248,-0.0101567628383621,
0.00144438106450357));
#47377=CARTESIAN_POINT('Ctrl Pts',(-0.00350715691927826,-0.0100388897777746,
0.00152470936290966));
#47378=CARTESIAN_POINT('Ctrl Pts',(-0.00351492312492403,-0.0099210167171871,
0.00160503766131575));
#47379=CARTESIAN_POINT('Ctrl Pts',(-0.0035210685455935,-0.00980324920461495,
0.00166556629660723));
#47380=CARTESIAN_POINT('Ctrl Pts',(-0.00352613224855201,-0.00968880590963078,
0.00171162816198026));
#47381=CARTESIAN_POINT('Ctrl Pts',(-0.00353625965446902,-0.00945991931966244,
0.00180375189272631));
#47382=CARTESIAN_POINT('Ctrl Pts',(-0.00354206018954218,-0.00924486720432927,
0.00183852795183029));
#47383=CARTESIAN_POINT('Ctrl Pts',(-0.00354305136176962,-0.00905532986970067,
0.00184421517727053));
#47384=CARTESIAN_POINT('Ctrl Pts',(-0.00354314889548398,-0.00903667894330822,
0.00184477481383644));
#47385=CARTESIAN_POINT('Ctrl Pts',(-0.00354319985999355,-0.00901827657119821,
0.00184507818656813));
#47386=CARTESIAN_POINT('Ctrl Pts',(-0.00354320482548136,-0.00900000021011351,
0.00184504509674603));
#47387=CARTESIAN_POINT('',(-0.00351041058117098,-0.00998279412709383,-0.00156095906068015));
#47388=CARTESIAN_POINT('Ctrl Pts',(-0.00351041058117098,-0.00998279412709383,
-0.00156095906068015));
#47389=CARTESIAN_POINT('Ctrl Pts',(-0.00350503565073693,-0.0100712857860722,
-0.00150479333735148));
#47390=CARTESIAN_POINT('Ctrl Pts',(-0.00349908543560267,-0.0101583121039841,
-0.00143987313134139));
#47391=CARTESIAN_POINT('Ctrl Pts',(-0.00349265305418288,-0.0102406671409818,
-0.00136503525702602));
#47392=CARTESIAN_POINT('Ctrl Pts',(-0.00348415640625082,-0.0103494513857482,
-0.0012661805672085));
#47393=CARTESIAN_POINT('Ctrl Pts',(-0.0034748184629296,-0.010449817819995,
-0.00114927353402808));
#47394=CARTESIAN_POINT('Ctrl Pts',(-0.00346709473226563,-0.010529157575455,
-0.00103170790983867));
#47395=CARTESIAN_POINT('Ctrl Pts',(-0.00345937100160166,-0.0106084973309151,
-0.000914142285649252));
#47396=CARTESIAN_POINT('Ctrl Pts',(-0.00345326148359495,-0.0106682116915477,
-0.000796826453053891));
#47397=CARTESIAN_POINT('Ctrl Pts',(-0.00344822616196539,-0.0107135768056789,
-0.00068306236416258));
#47398=CARTESIAN_POINT('Ctrl Pts',(-0.00343815551870626,-0.0108043070339414,
-0.000455534186379958));
#47399=CARTESIAN_POINT('Ctrl Pts',(-0.00343238166095573,-0.010838317159131,
-0.000242698364579505));
#47400=CARTESIAN_POINT('Ctrl Pts',(-0.0034313904685574,-0.010843958746556,
-5.52436125775062E-5));
#47401=CARTESIAN_POINT('Ctrl Pts',(-0.00343089369236729,-0.010846786256444,
3.87069238425434E-5));
#47402=CARTESIAN_POINT('Ctrl Pts',(-0.0034315982829426,-0.0108431244209408,
0.000126235007852828));
#47403=CARTESIAN_POINT('Ctrl Pts',(-0.0034334326877276,-0.0108311652892733,
0.000224075842000479));
#47404=CARTESIAN_POINT('Ctrl Pts',(-0.00343526709251259,-0.0108192061576057,
0.00032191667614813));
#47405=CARTESIAN_POINT('Ctrl Pts',(-0.00343823131150726,-0.0107979583547719,
0.00042991273046499));
#47406=CARTESIAN_POINT('Ctrl Pts',(-0.00344246340899626,-0.0107631486692495,
0.000542994992638243));
#47407=CARTESIAN_POINT('Ctrl Pts',(-0.00344767087270343,-0.0107203164390168,
0.000682139182421738));
#47408=CARTESIAN_POINT('Ctrl Pts',(-0.00345479797208566,-0.0106564757789345,
0.000828721308141272));
#47409=CARTESIAN_POINT('Ctrl Pts',(-0.0034634765427239,-0.0105683977214321,
0.000971535379578606));
#47410=CARTESIAN_POINT('',(-0.00354320118263476,-0.00900000021011351,-0.00184454176892424));
#47411=CARTESIAN_POINT('Ctrl Pts',(-0.00354320118263475,-0.00900000021011351,
-0.00184454176892423));
#47412=CARTESIAN_POINT('Ctrl Pts',(-0.00354322235846656,-0.00918058010367667,
-0.00184454176892423));
#47413=CARTESIAN_POINT('Ctrl Pts',(-0.0035391615244012,-0.00936903830252743,
-0.00182124852647729));
#47414=CARTESIAN_POINT('Ctrl Pts',(-0.00353056522115507,-0.00958285903313648,
-0.00175004499730282));
#47415=CARTESIAN_POINT('Ctrl Pts',(-0.00352538552624717,-0.00971169652500126,
-0.00170714137385795));
#47416=CARTESIAN_POINT('Ctrl Pts',(-0.00351855915924712,-0.00984886947693798,
-0.00164452038017344));
#47417=CARTESIAN_POINT('Ctrl Pts',(-0.00351041058117098,-0.00998279412709383,
-0.00156095906068015));
#47418=CARTESIAN_POINT('',(-0.00344269829706477,-0.00899998224949465,-0.0019508416734421));
#47419=CARTESIAN_POINT('Ctrl Pts',(-0.0035430763752057,-0.00899997871652083,
-0.00183940200010974));
#47420=CARTESIAN_POINT('Ctrl Pts',(-0.00343036413387564,-0.00900359568068924,
-0.00184212383138552));
#47421=CARTESIAN_POINT('Ctrl Pts',(-0.00344269760915441,-0.00899966251490034,
-0.00195083018299261));
#47422=CARTESIAN_POINT('Ctrl Pts',(-0.00343811948343117,-0.00856602524158671,
-0.00190328650635992));
#47423=CARTESIAN_POINT('Ctrl Pts',(-0.00342588491711595,-0.00806991020548021,
-0.00178978411271727));
#47424=CARTESIAN_POINT('Ctrl Pts',(-0.00338833186763894,-0.0076211810804679,
-0.00147075499299911));
#47425=CARTESIAN_POINT('Ctrl Pts',(-0.00336304853230225,-0.00735085164113558,
-0.0010394704028618));
#47426=CARTESIAN_POINT('Ctrl Pts',(-0.00333770359226152,-0.007079863524264,
-0.000607134956135401));
#47427=CARTESIAN_POINT('Ctrl Pts',(-0.00332461392794817,-0.00698753194456297,
-6.19190052309529E-5));
#47428=CARTESIAN_POINT('Ctrl Pts',(-0.00333682039814131,-0.00710081857461815,
0.000435571842955638));
#47429=CARTESIAN_POINT('Ctrl Pts',(-0.00334902702020896,-0.0072141066142004,
0.00093306888098847));
#47430=CARTESIAN_POINT('Ctrl Pts',(-0.00338655269909503,-0.00753311840533425,
0.00138301292867687));
#47431=CARTESIAN_POINT('Ctrl Pts',(-0.00341190064738082,-0.00796439294659748,
0.00165407866047813));
#47432=CARTESIAN_POINT('Ctrl Pts',(-0.00343719647682001,-0.008394780728451,
0.00192458704408161));
#47433=CARTESIAN_POINT('Ctrl Pts',(-0.0034503670171907,-0.00893739172396015,
0.00201689158354413));
#47434=CARTESIAN_POINT('Ctrl Pts',(-0.00343812749401439,-0.00943381877923568,
0.0019033576050533));
#47435=CARTESIAN_POINT('Ctrl Pts',(-0.0034258863648898,-0.00993031097072339,
0.00178980872976497));
#47436=CARTESIAN_POINT('Ctrl Pts',(-0.00338827163289001,-0.0103792185588139,
0.00147031465433104));
#47437=CARTESIAN_POINT('Ctrl Pts',(-0.00336301754592899,-0.0106492742069023,
0.00103896446141111));
#47438=CARTESIAN_POINT('Ctrl Pts',(-0.00333768686130201,-0.0109201489553746,
0.000606305948849976));
#47439=CARTESIAN_POINT('Ctrl Pts',(-0.00332462452155332,-0.0110126317008106,
6.0649363322396E-5));
#47440=CARTESIAN_POINT('Ctrl Pts',(-0.0033368677474717,-0.0108989627167492,
-0.000437415336783552));
#47441=CARTESIAN_POINT('Ctrl Pts',(-0.00334908127026236,-0.0107855695034998,
-0.000934271688738113));
#47442=CARTESIAN_POINT('Ctrl Pts',(-0.00338659264096821,-0.0104663958268669,
-0.00138368266598467));
#47443=CARTESIAN_POINT('Ctrl Pts',(-0.00341194350505705,-0.0100347423930322,
-0.00165451698700712));
#47444=CARTESIAN_POINT('Ctrl Pts',(-0.00342998476581804,-0.00972755080654826,
-0.00184725963244392));
#47445=CARTESIAN_POINT('Ctrl Pts',(-0.00344182965882166,-0.00936349053257669,
-0.00194935387765926));
#47446=CARTESIAN_POINT('Ctrl Pts',(-0.00344269801735234,-0.00900009946290338,
-0.00195084119718763));
#47447=CARTESIAN_POINT('Ctrl Pts',(-0.00344269811071666,-0.00900006039175898,
-0.00195084135710151));
#47448=CARTESIAN_POINT('Ctrl Pts',(-0.00344269820395414,-0.00900002132062265,
-0.001950841515853));
#47449=CARTESIAN_POINT('Ctrl Pts',(-0.00344269829706477,-0.00899998224949465,
-0.0019508416734421));
#47450=CARTESIAN_POINT('Ctrl Pts',(-0.00326780102756652,-0.00830776627881815,
-0.0010397814251779));
#47451=CARTESIAN_POINT('Ctrl Pts',(-0.0033697381364207,-0.00830650974827726,
-0.00103678809623668));
#47452=CARTESIAN_POINT('Ctrl Pts',(-0.00336771328390501,-0.00824815804099986,
-0.00112260420442851));
#47453=CARTESIAN_POINT('Ctrl Pts',(-0.00326464920350823,-0.00823890453247449,
-0.000994386776895733));
#47454=CARTESIAN_POINT('Ctrl Pts',(-0.00336706234466192,-0.00823684759055849,
-0.000991078081392678));
#47455=CARTESIAN_POINT('Ctrl Pts',(-0.0033645459846626,-0.00817342874147058,
-0.00107361247034106));
#47456=CARTESIAN_POINT('Ctrl Pts',(-0.00324793746847567,-0.00791953227740259,
-0.00073567091108549));
#47457=CARTESIAN_POINT('Ctrl Pts',(-0.00335277774940962,-0.00791087001891881,
-0.000729341170399936));
#47458=CARTESIAN_POINT('Ctrl Pts',(-0.00334776231449907,-0.00782709178377431,
-0.000794513134553083));
#47459=CARTESIAN_POINT('Ctrl Pts',(-0.00321793190913946,-0.0076149676140644,
-1.54083867402206E-6));
#47460=CARTESIAN_POINT('Ctrl Pts',(-0.00332799412930291,-0.00761878655976351,
-1.51388930652299E-6));
#47461=CARTESIAN_POINT('Ctrl Pts',(-0.00331757760893123,-0.00749558137023603,
-1.66483058764779E-6));
#47462=CARTESIAN_POINT('Ctrl Pts',(-0.00325780785275684,-0.008019466089899,
0.000978742800856142));
#47463=CARTESIAN_POINT('Ctrl Pts',(-0.00336067162260847,-0.00800363754489395,
0.000962724449561964));
#47464=CARTESIAN_POINT('Ctrl Pts',(-0.0033577150665097,-0.00793612611646283,
0.0010576437152649));
#47465=CARTESIAN_POINT('Ctrl Pts',(-0.00329800025932114,-0.00899946420378033,
0.00138546387197374));
#47466=CARTESIAN_POINT('Ctrl Pts',(-0.0033953190356324,-0.00899944782531834,
0.00138926904137042));
#47467=CARTESIAN_POINT('Ctrl Pts',(-0.00339807408715874,-0.00899941917617344,
0.00149541593485778));
#47468=CARTESIAN_POINT('Ctrl Pts',(-0.00325786406347626,-0.00997987109426551,
0.000979401186339539));
#47469=CARTESIAN_POINT('Ctrl Pts',(-0.00336071891445555,-0.00999571441285378,
0.000963399852332962));
#47470=CARTESIAN_POINT('Ctrl Pts',(-0.00335777157893346,-0.010063153048397,
0.00105835340798998));
#47471=CARTESIAN_POINT('Ctrl Pts',(-0.00321793255865113,-0.0103850227343342,
-4.38299481707064E-7));
#47472=CARTESIAN_POINT('Ctrl Pts',(-0.00332799471446149,-0.0103812033852223,
-4.47410730017003E-7));
#47473=CARTESIAN_POINT('Ctrl Pts',(-0.00331757825861524,-0.0105044081817788,
-4.72359875001561E-7));
#47474=CARTESIAN_POINT('Ctrl Pts',(-0.00325784210153424,-0.00998003788779652,
-0.000978747541355083));
#47475=CARTESIAN_POINT('Ctrl Pts',(-0.00336070043689,-0.00999586177973733,
-0.00096275163289535));
#47476=CARTESIAN_POINT('Ctrl Pts',(-0.00335774949912804,-0.0100633355839779,
-0.00105764734367712));
#47477=CARTESIAN_POINT('Ctrl Pts',(-0.00328460231345262,-0.00932704381043793,
-0.00124988324087735));
#47478=CARTESIAN_POINT('Ctrl Pts',(-0.00338399728153908,-0.00932579560598706,
-0.00124988491617768));
#47479=CARTESIAN_POINT('Ctrl Pts',(-0.00338460037758513,-0.00935537209178598,
-0.00134926500141788));
#47480=CARTESIAN_POINT('Ctrl Pts',(-0.00328461215845628,-0.00900048192889801,
-0.00124999990709781));
#47481=CARTESIAN_POINT('Ctrl Pts',(-0.00338400522957233,-0.00900048496365769,
-0.00124999990592778));
#47482=CARTESIAN_POINT('Ctrl Pts',(-0.00338461030538419,-0.00900052330173693,
-0.00134939112791716));
#47483=CARTESIAN_POINT('Ctrl Pts',(-0.003284619521066,-0.00875626183863264,
-0.001250087156212));
#47484=CARTESIAN_POINT('Ctrl Pts',(-0.0033840111734513,-0.00875720376069227,
-0.00125008590017788));
#47485=CARTESIAN_POINT('Ctrl Pts',(-0.00338461772991996,-0.00873514851728435,
-0.00134948545201661));
#47486=CARTESIAN_POINT('Ctrl Pts',(-0.0032771491209721,-0.00851200548284287,
-0.00117441883018739));
#47487=CARTESIAN_POINT('Ctrl Pts',(-0.00337760001855469,-0.00851118773616096,
-0.00117109105455409));
#47488=CARTESIAN_POINT('Ctrl Pts',(-0.00337711394211846,-0.0084699572931819,
-0.00126801343550846));
#47489=CARTESIAN_POINT('Ctrl Pts',(-0.00326780102756652,-0.00830776627881815,
-0.0010397814251779));
#47490=CARTESIAN_POINT('Ctrl Pts',(-0.0033697381364207,-0.00830650974827726,
-0.00103678809623668));
#47491=CARTESIAN_POINT('Ctrl Pts',(-0.00336771328390501,-0.00824815804099986,
-0.00112260420442851));
#47492=CARTESIAN_POINT('',(-0.00338450873183093,-0.00900052178030338,-0.00134545296373893));
#47493=CARTESIAN_POINT('',(-0.00328461216640222,-0.00900000000000097,-0.00124999998094225));
#47494=CARTESIAN_POINT('Ctrl Pts',(-0.00338450873198576,-0.0090005217803047,
-0.00134545296714054));
#47495=CARTESIAN_POINT('Ctrl Pts',(-0.00338016405263189,-0.00900048484637538,
-0.001249999905973));
#47496=CARTESIAN_POINT('Ctrl Pts',(-0.00328461215845628,-0.00900048192889801,
-0.00124999990709781));
#47497=CARTESIAN_POINT('',(-0.00336798809794631,-0.00974865428221822,-0.00111800482524904));
#47498=CARTESIAN_POINT('Ctrl Pts',(-0.00338450873183093,-0.00900052178030331,
-0.00134545296373893));
#47499=CARTESIAN_POINT('Ctrl Pts',(-0.00338450865110421,-0.00900327476401382,
-0.00134545189664552));
#47500=CARTESIAN_POINT('Ctrl Pts',(-0.00338450777831145,-0.00900602772712384,
-0.00134544238252916));
#47501=CARTESIAN_POINT('Ctrl Pts',(-0.00338450330004073,-0.00901345676316639,
-0.0013453939127586));
#47502=CARTESIAN_POINT('Ctrl Pts',(-0.00338449821153448,-0.00901813267771828,
-0.00134533903309341));
#47503=CARTESIAN_POINT('Ctrl Pts',(-0.00338444973233171,-0.00904904765956048,
-0.00134481503658746));
#47504=CARTESIAN_POINT('Ctrl Pts',(-0.00338433794923329,-0.00907526822596815,
-0.00134360289963365));
#47505=CARTESIAN_POINT('Ctrl Pts',(-0.00338369809843344,-0.0091694579286069,
-0.00133648353622328));
#47506=CARTESIAN_POINT('Ctrl Pts',(-0.00338279100650046,-0.00923698523823002,
-0.00132617824733123));
#47507=CARTESIAN_POINT('Ctrl Pts',(-0.00338117494196493,-0.00932185601914471,
-0.00130653740876165));
#47508=CARTESIAN_POINT('Ctrl Pts',(-0.00338079683170026,-0.00934018495676536,
-0.00130188671281531));
#47509=CARTESIAN_POINT('Ctrl Pts',(-0.00338022254096741,-0.00936612142649954,
-0.00129472079666794));
#47510=CARTESIAN_POINT('Ctrl Pts',(-0.00338004723694626,-0.00937381430467724,
-0.00129252132910337));
#47511=CARTESIAN_POINT('Ctrl Pts',(-0.00337853814796015,-0.0094382488903721,
-0.00127347571440452));
#47512=CARTESIAN_POINT('Ctrl Pts',(-0.00337697029016163,-0.00949383715135224,
-0.00125297317161244));
#47513=CARTESIAN_POINT('Ctrl Pts',(-0.00337295941941667,-0.00961784810662058,
-0.00119770077189597));
#47514=CARTESIAN_POINT('Ctrl Pts',(-0.00337040139297908,-0.0096850095454096,
-0.00116060817391342));
#47515=CARTESIAN_POINT('Ctrl Pts',(-0.0033676724655748,-0.00974864493507495,
-0.00111801108221903));
#47516=CARTESIAN_POINT('',(-0.00335782220510489,-0.00995293472304761,-0.000949979974017949));
#47517=CARTESIAN_POINT('Origin',(-0.00336290519953541,-0.00899804839933691,
2.75513276777065E-6));
#47518=CARTESIAN_POINT('',(-0.0033395154778931,-0.0102443751187985,0.000513026049606027));
#47519=CARTESIAN_POINT('Ctrl Pts',(-0.00333951547892669,-0.0102443751214304,
0.000513026050658624));
#47520=CARTESIAN_POINT('Ctrl Pts',(-0.00333720158736698,-0.0102754775655337,
0.00043752897741956));
#47521=CARTESIAN_POINT('Ctrl Pts',(-0.00333524185476234,-0.0102996487655498,
0.000359348111851545));
#47522=CARTESIAN_POINT('Ctrl Pts',(-0.00333219371656032,-0.0103353522363518,
0.000190907331342745));
#47523=CARTESIAN_POINT('Ctrl Pts',(-0.00333122867855846,-0.0103451419971487,
0.000100686070978564));
#47524=CARTESIAN_POINT('Ctrl Pts',(-0.00333114619591799,-0.0103458982369924,
-3.36368651573786E-6));
#47525=CARTESIAN_POINT('Ctrl Pts',(-0.00333115576494018,-0.0103457925958847,
-1.68909191838913E-5));
#47526=CARTESIAN_POINT('Ctrl Pts',(-0.00333120143442851,-0.0103453098793274,
-3.79805317566844E-5));
#47527=CARTESIAN_POINT('Ctrl Pts',(-0.00333122396405323,-0.010345072876226,
-4.5545203362486E-5));
#47528=CARTESIAN_POINT('Ctrl Pts',(-0.00333134781289938,-0.010343766788362,
-7.83812280955537E-5));
#47529=CARTESIAN_POINT('Ctrl Pts',(-0.00333151003988135,-0.010342049212991,
-0.000103621277838774));
#47530=CARTESIAN_POINT('Ctrl Pts',(-0.00333213219199593,-0.0103352897395069,
-0.000173718461075599));
#47531=CARTESIAN_POINT('Ctrl Pts',(-0.00333272515882828,-0.0103287014280872,
-0.000218391262500524));
#47532=CARTESIAN_POINT('Ctrl Pts',(-0.00333561490513267,-0.0102950073937465,
-0.000387468756320592));
#47533=CARTESIAN_POINT('Ctrl Pts',(-0.00333902150429297,-0.0102525546405954,
-0.000508114028806056));
#47534=CARTESIAN_POINT('Ctrl Pts',(-0.00334530384177048,-0.010162122328243,
-0.000681861044479222));
#47535=CARTESIAN_POINT('Ctrl Pts',(-0.00334769471416655,-0.0101258236197889,
-0.000740228332633532));
#47536=CARTESIAN_POINT('Ctrl Pts',(-0.00335265664561079,-0.010045090781357,
-0.000850303231101744));
#47537=CARTESIAN_POINT('Ctrl Pts',(-0.00335521909692295,-0.0100008637934157,
-0.000901921239805929));
#47538=CARTESIAN_POINT('Ctrl Pts',(-0.00335779790172574,-0.00995293407100622,
-0.000949980627823781));
#47539=CARTESIAN_POINT('',(-0.00338454060301105,-0.00900002810628826,0.00134621762248316));
#47540=CARTESIAN_POINT('Ctrl Pts',(-0.00338454060675955,-0.0090000281062885,
0.00134621763156711));
#47541=CARTESIAN_POINT('Ctrl Pts',(-0.00338454054544131,-0.00900662374474969,
0.00134621749439546));
#47542=CARTESIAN_POINT('Ctrl Pts',(-0.00338453591899628,-0.00901321923754373,
0.0013461688717259));
#47543=CARTESIAN_POINT('Ctrl Pts',(-0.00338451628347078,-0.00902742516719074,
0.00134595970333058));
#47544=CARTESIAN_POINT('Ctrl Pts',(-0.00338449978460471,-0.00903503515915829,
0.00134578306823355));
#47545=CARTESIAN_POINT('Ctrl Pts',(-0.00338443289937514,-0.00905779189537234,
0.00134506165343333));
#47546=CARTESIAN_POINT('Ctrl Pts',(-0.00338436513907917,-0.00907293127221901,
0.00134432556283098));
#47547=CARTESIAN_POINT('Ctrl Pts',(-0.00338409618593173,-0.0091180888868096,
0.00134136466489044));
#47548=CARTESIAN_POINT('Ctrl Pts',(-0.00338382938092011,-0.00914804765314941,
0.00133838846566736));
#47549=CARTESIAN_POINT('Ctrl Pts',(-0.00338278037558188,-0.00923814805753341,
0.0013263743961517));
#47550=CARTESIAN_POINT('Ctrl Pts',(-0.00338175141220183,-0.00929779697665544,
0.00131426408186406));
#47551=CARTESIAN_POINT('Ctrl Pts',(-0.00338028716191064,-0.00936421426237214,
0.00129602352001954));
#47552=CARTESIAN_POINT('Ctrl Pts',(-0.0033801106422181,-0.00937199137910707,
0.00129381208644705));
#47553=CARTESIAN_POINT('Ctrl Pts',(-0.00337973723180336,-0.00938799351482061,
0.00128910559654723));
#47554=CARTESIAN_POINT('Ctrl Pts',(-0.00337953976697067,-0.00939621550146254,
0.00128660155700354));
#47555=CARTESIAN_POINT('Ctrl Pts',(-0.00337872702498143,-0.00942914195675233,
0.00127622800099797));
#47556=CARTESIAN_POINT('Ctrl Pts',(-0.0033780724469702,-0.0094536398055474,
0.00126772435961022));
#47557=CARTESIAN_POINT('Ctrl Pts',(-0.00337621160674814,-0.00951863915914454,
0.00124303578009676));
#47558=CARTESIAN_POINT('Ctrl Pts',(-0.00337493469975409,-0.00955862344005493,
0.00122558171909746));
#47559=CARTESIAN_POINT('Ctrl Pts',(-0.00337148711508259,-0.0096573552598843,
0.00117664413953565));
#47560=CARTESIAN_POINT('Ctrl Pts',(-0.00336920456265393,-0.0097147409601528,
0.00114268340946798));
#47561=CARTESIAN_POINT('Ctrl Pts',(-0.00336263194246688,-0.00986438322421787,
0.00103842072052163));
#47562=CARTESIAN_POINT('Ctrl Pts',(-0.00335813345016562,-0.00995045109400686,
0.000960238410779958));
#47563=CARTESIAN_POINT('Ctrl Pts',(-0.0033511420936047,-0.0100714232924326,
0.000817918363258607));
#47564=CARTESIAN_POINT('Ctrl Pts',(-0.00334855089328028,-0.0101130526115715,
0.000760269195348086));
#47565=CARTESIAN_POINT('Ctrl Pts',(-0.00334372576596367,-0.0101862077048872,
0.000639957996819968));
#47566=CARTESIAN_POINT('Ctrl Pts',(-0.00334149390895866,-0.0102177818226984,
0.000577577769343556));
#47567=CARTESIAN_POINT('Ctrl Pts',(-0.00333951547892579,-0.0102443751214424,
0.000513026050629553));
#47568=CARTESIAN_POINT('',(-0.00333951973713618,-0.00775564716847025,0.0005130795639787));
#47569=CARTESIAN_POINT('Ctrl Pts',(-0.00333951974170471,-0.00775564716011877,
0.000513079567279669));
#47570=CARTESIAN_POINT('Ctrl Pts',(-0.00334149417117988,-0.00778219525425979,
0.000577513689473508));
#47571=CARTESIAN_POINT('Ctrl Pts',(-0.00334372094979989,-0.00781370628872191,
0.000639784345303221));
#47572=CARTESIAN_POINT('Ctrl Pts',(-0.00334854033125506,-0.00788678174994642,
0.000760028693420967));
#47573=CARTESIAN_POINT('Ctrl Pts',(-0.00335113155174353,-0.00792841497623692,
0.000817708394398717));
#47574=CARTESIAN_POINT('Ctrl Pts',(-0.00335812613437231,-0.00804944390357773,
0.000960146213641191));
#47575=CARTESIAN_POINT('Ctrl Pts',(-0.00336262891395931,-0.00813558116512314,
0.00103840197563686));
#47576=CARTESIAN_POINT('Ctrl Pts',(-0.00336914360363133,-0.00828388637151784,
0.00114172335762287));
#47577=CARTESIAN_POINT('Ctrl Pts',(-0.00337137024002632,-0.0083397105219415,
0.00117490230676323));
#47578=CARTESIAN_POINT('Ctrl Pts',(-0.00337479463125309,-0.00843708313587216,
0.001223630170499));
#47579=CARTESIAN_POINT('Ctrl Pts',(-0.00337609125760534,-0.00847739854758708,
0.0012413895470228));
#47580=CARTESIAN_POINT('Ctrl Pts',(-0.00337798033922486,-0.00854293077009745,
0.0012664960464477));
#47581=CARTESIAN_POINT('Ctrl Pts',(-0.00337864447915115,-0.00856761559147129,
0.00127513723333758));
#47582=CARTESIAN_POINT('Ctrl Pts',(-0.00337946877993396,-0.00860078220827126,
0.00128567317765247));
#47583=CARTESIAN_POINT('Ctrl Pts',(-0.00337966877160793,-0.00860905215495234,
0.00128821275223784));
#47584=CARTESIAN_POINT('Ctrl Pts',(-0.00338023165440961,-0.00863300704057187,
0.00129531691606092));
#47585=CARTESIAN_POINT('Ctrl Pts',(-0.00338058140838721,-0.00864875161229656,
0.00129967598971537));
#47586=CARTESIAN_POINT('Ctrl Pts',(-0.00338206491416227,-0.0087198150702577,
0.00131796455658876));
#47587=CARTESIAN_POINT('Ctrl Pts',(-0.00338297907469519,-0.00877591025581751,
0.00132865611872142));
#47588=CARTESIAN_POINT('Ctrl Pts',(-0.00338391060684845,-0.00886062949802715,
0.00133928156763364));
#47589=CARTESIAN_POINT('Ctrl Pts',(-0.00338414750987857,-0.00888884576435987,
0.00134191880644743));
#47590=CARTESIAN_POINT('Ctrl Pts',(-0.00338438590382474,-0.00893136516583988,
0.00134454209115992));
#47591=CARTESIAN_POINT('Ctrl Pts',(-0.00338444586200037,-0.00894561869572669,
0.00134519417029263));
#47592=CARTESIAN_POINT('Ctrl Pts',(-0.00338450489567835,-0.00896703848358398,
0.00134583299070457));
#47593=CARTESIAN_POINT('Ctrl Pts',(-0.00338451941982857,-0.00897419859695921,
0.00134598934228585));
#47594=CARTESIAN_POINT('Ctrl Pts',(-0.00338453325841651,-0.00898494452379937,
0.00134613819300853));
#47595=CARTESIAN_POINT('Ctrl Pts',(-0.00338453654617301,-0.00898852960715314,
0.00134617352521678));
#47596=CARTESIAN_POINT('Ctrl Pts',(-0.00338453992474177,-0.0089947519580479,
0.00134620998295414));
#47597=CARTESIAN_POINT('Ctrl Pts',(-0.00338454063097428,-0.00899738915780249,
0.00134621768306205));
#47598=CARTESIAN_POINT('Ctrl Pts',(-0.00338454060677552,-0.00900002637780627,
0.00134621763160195));
#47599=CARTESIAN_POINT('',(-0.00335781975105043,-0.0080470214493883,-0.000949935792125509));
#47600=CARTESIAN_POINT('Ctrl Pts',(-0.00335779717912834,-0.00804702205697391,
-0.00094993640141179));
#47601=CARTESIAN_POINT('Ctrl Pts',(-0.00335522018045496,-0.00799912930709866,
-0.000901909628323764));
#47602=CARTESIAN_POINT('Ctrl Pts',(-0.00335265916585628,-0.00795493403683286,
-0.000850329509246332));
#47603=CARTESIAN_POINT('Ctrl Pts',(-0.0033476987953991,-0.00787424156296798,
-0.000740324203404496));
#47604=CARTESIAN_POINT('Ctrl Pts',(-0.00334530809252378,-0.00783795350784308,
-0.000681986711934992));
#47605=CARTESIAN_POINT('Ctrl Pts',(-0.00333902318351723,-0.00774750315184934,
-0.000508260877900045));
#47606=CARTESIAN_POINT('Ctrl Pts',(-0.00333561409435754,-0.00770503036771147,
-0.000387600728429948));
#47607=CARTESIAN_POINT('Ctrl Pts',(-0.00333272868774576,-0.00767137842777274,
-0.000218810613518203));
#47608=CARTESIAN_POINT('Ctrl Pts',(-0.00333213872536355,-0.00766481632598804,
-0.000174448386311072));
#47609=CARTESIAN_POINT('Ctrl Pts',(-0.00333151671899573,-0.00765804482743786,
-0.000104793834325934));
#47610=CARTESIAN_POINT('Ctrl Pts',(-0.00333135366625433,-0.00765631286321025,
-7.96840624127513E-5));
#47611=CARTESIAN_POINT('Ctrl Pts',(-0.00333122767584969,-0.00765497703325505,
-4.69777802509182E-5));
#47612=CARTESIAN_POINT('Ctrl Pts',(-0.00333120453567573,-0.00765473195936074,
-3.9412892698668E-5));
#47613=CARTESIAN_POINT('Ctrl Pts',(-0.00333118003267711,-0.00765447067095878,
-2.85048715363367E-5));
#47614=CARTESIAN_POINT('Ctrl Pts',(-0.0033311737247941,-0.00765440307861096,
-2.51631309465576E-5));
#47615=CARTESIAN_POINT('Ctrl Pts',(-0.00333115945419868,-0.00765424868323619,
-1.58059170859384E-5));
#47616=CARTESIAN_POINT('Ctrl Pts',(-0.00333115420416645,-0.00765418976528437,
-9.79006205307497E-6));
#47617=CARTESIAN_POINT('Ctrl Pts',(-0.00333113514184231,-0.00765390670655867,
8.18657661644229E-5));
#47618=CARTESIAN_POINT('Ctrl Pts',(-0.00333192890168699,-0.00766181744535084,
0.000167330559431246));
#47619=CARTESIAN_POINT('Ctrl Pts',(-0.0033347928732721,-0.00769481203868999,
0.00034108911925425));
#47620=CARTESIAN_POINT('Ctrl Pts',(-0.0033369356378662,-0.00772090137562988,
0.000428749383032905));
#47621=CARTESIAN_POINT('Ctrl Pts',(-0.00333951979241417,-0.00775564784195628,
0.00051308122214492));
#47622=CARTESIAN_POINT('',(-0.00336798575526351,-0.00825128999511177,-0.0011179673661904));
#47623=CARTESIAN_POINT('Origin',(-0.00336290275316926,-0.00900195197300184,
2.75506903634454E-6));
#47624=CARTESIAN_POINT('',(-0.00326780067323885,-0.00830775851653247,-0.00103977630810674));
#47625=CARTESIAN_POINT('Ctrl Pts',(-0.0033676712709598,-0.00825129322272922,
-0.00111798268825413));
#47626=CARTESIAN_POINT('Ctrl Pts',(-0.00336429022081308,-0.00830656906493108,
-0.00103694292107723));
#47627=CARTESIAN_POINT('Ctrl Pts',(-0.00326780067212508,-0.00830775851309429,
-0.00103977630586051));
#47628=CARTESIAN_POINT('',(-0.00325791983579602,-0.00811636346334185,-0.000884130347337319));
#47629=CARTESIAN_POINT('Ctrl Pts',(-0.00325791983579602,-0.00811636346334185,
-0.000884130347337319));
#47630=CARTESIAN_POINT('Ctrl Pts',(-0.00326128379583907,-0.0081745896155171,
-0.000942286360207792));
#47631=CARTESIAN_POINT('Ctrl Pts',(-0.00326464894774107,-0.00823889962784297,
-0.000994382814554614));
#47632=CARTESIAN_POINT('Ctrl Pts',(-0.00326780067323886,-0.00830775851653247,
-0.00103977630810674));
#47633=CARTESIAN_POINT('',(-0.003257865684124,-0.00811545508239479,0.000883221550452495));
#47634=CARTESIAN_POINT('Ctrl Pts',(-0.003257865684124,-0.00811545508239479,
0.000883221550452495));
#47635=CARTESIAN_POINT('Ctrl Pts',(-0.00324452625828876,-0.00788477670656564,
0.000652165360404284));
#47636=CARTESIAN_POINT('Ctrl Pts',(-0.00323123706542317,-0.00774993409998482,
0.000325577072709837));
#47637=CARTESIAN_POINT('Ctrl Pts',(-0.00323124079846264,-0.0077500003261204,
-6.59450910766848E-7));
#47638=CARTESIAN_POINT('Ctrl Pts',(-0.00323124453297722,-0.00775006657842525,
-0.000327024886920311));
#47639=CARTESIAN_POINT('Ctrl Pts',(-0.00324455815677214,-0.00788518359895288,
-0.000653038877261263));
#47640=CARTESIAN_POINT('Ctrl Pts',(-0.00325789992482187,-0.00811601889883439,
-0.000883786056135089));
#47641=CARTESIAN_POINT('',(-0.00328461358329975,-0.00900001820654589,0.00124999997585377));
#47642=CARTESIAN_POINT('Ctrl Pts',(-0.00328461358329975,-0.00900001820654589,
0.00124999997585377));
#47643=CARTESIAN_POINT('Ctrl Pts',(-0.00328461606383265,-0.00867328446293999,
0.00125002453056291));
#47644=CARTESIAN_POINT('Ctrl Pts',(-0.00327122623192912,-0.00834657387630014,
0.00111456735937024));
#47645=CARTESIAN_POINT('Ctrl Pts',(-0.00325788149737239,-0.00811572858503246,
0.000883495411303269));
#47646=CARTESIAN_POINT('',(-0.00325789817864836,-0.00988399521919616,0.000883771719641636));
#47647=CARTESIAN_POINT('Ctrl Pts',(-0.00325789817864836,-0.00988399521919616,
0.000883771719641636));
#47648=CARTESIAN_POINT('Ctrl Pts',(-0.00327123613082152,-0.00965318416122461,
0.0011146399923813));
#47649=CARTESIAN_POINT('Ctrl Pts',(-0.00328461110399896,-0.00932658965853997,
0.00124997543334117));
#47650=CARTESIAN_POINT('Ctrl Pts',(-0.00328461358329975,-0.00900001820654589,
0.00124999997585377));
#47651=CARTESIAN_POINT('',(-0.00325788569625234,-0.00988421312102252,-0.000883553669847396));
#47652=CARTESIAN_POINT('Ctrl Pts',(-0.00325788569625234,-0.00988421312102252,
-0.000883553669847396));
#47653=CARTESIAN_POINT('Ctrl Pts',(-0.00324454916963038,-0.0101148915861028,
-0.000652826446188782));
#47654=CARTESIAN_POINT('Ctrl Pts',(-0.00323124877940481,-0.0102498954446246,
-0.000326895092343441));
#47655=CARTESIAN_POINT('Ctrl Pts',(-0.0032312407867353,-0.0102499999301743,
-6.63048329690229E-7));
#47656=CARTESIAN_POINT('Ctrl Pts',(-0.00323123279101768,-0.0102501044555711,
0.000325693408701394));
#47657=CARTESIAN_POINT('Ctrl Pts',(-0.00324453375313502,-0.0101151697465547,
0.000652349462123238));
#47658=CARTESIAN_POINT('Ctrl Pts',(-0.00325787829355509,-0.00988433925695948,
0.000883427454797046));
#47659=CARTESIAN_POINT('Ctrl Pts',(-0.00328461216640222,-0.00900000000000097,
-0.00124999998094225));
#47660=CARTESIAN_POINT('Ctrl Pts',(-0.00328461546930389,-0.00932656366198307,
-0.00125001656791605));
#47661=CARTESIAN_POINT('Ctrl Pts',(-0.00327124259279507,-0.00965310972898778,
-0.00111456015950205));
#47662=CARTESIAN_POINT('Ctrl Pts',(-0.00325790095446365,-0.00988394916218192,
-0.000883817601168605));
#47663=CARTESIAN_POINT('Origin',(2.6675363272169E-19,-0.002,0.));
#47664=CARTESIAN_POINT('',(0.0055,-0.002,-6.73555739531044E-19));
#47665=CARTESIAN_POINT('Origin',(2.6675363272169E-19,-0.002,0.));
#47666=CARTESIAN_POINT('',(0.0036018008897227,-0.002,0.00302090833547154));
#47667=CARTESIAN_POINT('',(0.00360180088972267,-0.002,-0.00302090833547154));
#47668=CARTESIAN_POINT('Origin',(0.0203312393987904,-0.002,-7.17008776061679E-17));
#47669=CARTESIAN_POINT('',(0.00302090833547152,-0.002,-0.00360180088972268));
#47670=CARTESIAN_POINT('Origin',(0.00310975858063245,-0.002,-0.00310975858063246));
#47671=CARTESIAN_POINT('',(-0.00302090833547157,-0.002,-0.00360180088972269));
#47672=CARTESIAN_POINT('Origin',(-4.47981017017182E-19,-0.002,-0.0203312393987904));
#47673=CARTESIAN_POINT('',(-0.00360180088972273,-0.002,-0.00302090833547154));
#47674=CARTESIAN_POINT('Origin',(-0.0031097585806325,-0.002,-0.00310975858063247));
#47675=CARTESIAN_POINT('',(-0.00360180088972265,-0.002,0.00302090833547154));
#47676=CARTESIAN_POINT('Origin',(-0.0203312393987904,-0.002,2.13673163519026E-16));
#47677=CARTESIAN_POINT('',(-0.00302090833547149,-0.002,0.00360180088972268));
#47678=CARTESIAN_POINT('Origin',(-0.00310975858063242,-0.002,0.00310975858063246));
#47679=CARTESIAN_POINT('',(0.00302090833547155,-0.002,0.00360180088972269));
#47680=CARTESIAN_POINT('Origin',(9.81488282460562E-19,-0.002,0.0203312393987904));
#47681=CARTESIAN_POINT('Origin',(0.00310975858063248,-0.002,0.00310975858063246));
#47682=CARTESIAN_POINT('Origin',(2.6675363272169E-19,-0.002,0.));
#47683=CARTESIAN_POINT('',(0.0055,0.014,-6.73555739531044E-19));
#47684=CARTESIAN_POINT('Origin',(-1.86727542905182E-18,0.014,0.));
#47685=CARTESIAN_POINT('',(0.0055,-0.002,-6.73555739531044E-19));
#47686=CARTESIAN_POINT('Origin',(-2.00065224541267E-18,0.015,0.));
#47687=CARTESIAN_POINT('',(0.0045,0.015,-5.51091059616309E-19));
#47688=CARTESIAN_POINT('Origin',(-2.00065224541267E-18,0.015,0.));
#47689=CARTESIAN_POINT('Origin',(1.96519507615456E-18,-0.015,0.));
#47690=CARTESIAN_POINT('',(-0.00360180088972265,-0.015,0.00302090833547154));
#47691=CARTESIAN_POINT('',(-0.00360180088972272,-0.015,-0.00302090833547154));
#47692=CARTESIAN_POINT('Origin',(-0.0203312393987904,-0.015,2.13126180968845E-16));
#47693=CARTESIAN_POINT('',(-0.00302090833547157,-0.015,-0.00360180088972269));
#47694=CARTESIAN_POINT('Origin',(-0.0031097585806325,-0.015,-0.00310975858063247));
#47695=CARTESIAN_POINT('',(0.00302090833547153,-0.015,-0.00360180088972268));
#47696=CARTESIAN_POINT('Origin',(1.83290014585433E-18,-0.015,-0.0203312393987904));
#47697=CARTESIAN_POINT('',(0.00360180088972268,-0.015,-0.00302090833547154));
#47698=CARTESIAN_POINT('Origin',(0.00310975858063245,-0.015,-0.00310975858063246));
#47699=CARTESIAN_POINT('',(0.0036018008897227,-0.015,0.00302090833547154));
#47700=CARTESIAN_POINT('Origin',(0.0203312393987904,-0.015,-7.11538950559874E-17));
#47701=CARTESIAN_POINT('',(0.00302090833547155,-0.015,0.00360180088972269));
#47702=CARTESIAN_POINT('Origin',(0.00310975858063248,-0.015,0.00310975858063246));
#47703=CARTESIAN_POINT('',(-0.00302090833547149,-0.015,0.00360180088972268));
#47704=CARTESIAN_POINT('Origin',(2.16840434497101E-18,-0.015,0.0203312393987904));
#47705=CARTESIAN_POINT('Origin',(-0.00310975858063242,-0.015,0.00310975858063246));
#47706=CARTESIAN_POINT('',(0.00278445714771808,-0.015,0.));
#47707=CARTESIAN_POINT('Origin',(1.7347234759768E-18,-0.015,0.));
#47708=CARTESIAN_POINT('Origin',(3.08141670074827E-18,-0.025,0.0203312393987904));
#47709=CARTESIAN_POINT('',(0.00302090833547155,-0.025,0.00360180088972269));
#47710=CARTESIAN_POINT('',(-0.00302090833547149,-0.025,0.00360180088972268));
#47711=CARTESIAN_POINT('Origin',(-0.0203312393987904,-0.025,2.12705425161014E-16));
#47712=CARTESIAN_POINT('',(-0.00360180088972272,-0.025,-0.00302090833547154));
#47713=CARTESIAN_POINT('',(-0.00360180088972265,-0.025,0.00302090833547154));
#47714=CARTESIAN_POINT('Ctrl Pts',(-0.00344269829706477,-0.00899998224949465,
-0.0019508416734421));
#47715=CARTESIAN_POINT('Ctrl Pts',(-0.00344304626547968,-0.00885396756551811,
-0.00195143060758549));
#47716=CARTESIAN_POINT('Ctrl Pts',(-0.00344162236167648,-0.00870806791987832,
-0.00193578337263521));
#47717=CARTESIAN_POINT('Ctrl Pts',(-0.00343811948343117,-0.00856602524158671,
-0.00190328650635992));
#47718=CARTESIAN_POINT('Origin',(0.0203312393987904,-0.025,-7.07331392481562E-17));
#47719=CARTESIAN_POINT('',(0.00360180088972268,-0.025,-0.00302090833547154));
#47720=CARTESIAN_POINT('',(0.0036018008897227,-0.025,0.00302090833547154));
#47721=CARTESIAN_POINT('Origin',(3.58742411729397E-18,-0.025,-0.0203312393987904));
#47722=CARTESIAN_POINT('',(-0.00302090833547157,-0.025,-0.00360180088972269));
#47723=CARTESIAN_POINT('',(0.00302090833547153,-0.025,-0.00360180088972268));
#47724=CARTESIAN_POINT('Origin',(-0.0031097585806325,-0.025,-0.00310975858063247));
#47725=CARTESIAN_POINT('Origin',(0.00310975858063245,-0.025,-0.00310975858063246));
#47726=CARTESIAN_POINT('Origin',(0.00310975858063248,-0.025,0.00310975858063246));
#47727=CARTESIAN_POINT('Origin',(-0.00310975858063242,-0.025,0.00310975858063246));
#47728=CARTESIAN_POINT('Origin',(1.76941794549634E-18,-0.0153,0.));
#47729=CARTESIAN_POINT('',(0.00278445714771808,-0.0152,0.));
#47730=CARTESIAN_POINT('',(0.00278445714771807,-0.0153,-3.4099765333159E-19));
#47731=CARTESIAN_POINT('',(-0.00278445714771807,-0.0152,-3.4099765333159E-19));
#47732=CARTESIAN_POINT('Origin',(1.75785312232316E-18,-0.0152,0.));
#47733=CARTESIAN_POINT('Origin',(1.75785312232316E-18,-0.0152,0.));
#47734=CARTESIAN_POINT('Origin',(1.76941794549634E-18,-0.0153,0.));
#47735=CARTESIAN_POINT('',(-0.00268445714771808,-0.0153,-3.28751185340118E-19));
#47736=CARTESIAN_POINT('Origin',(1.76941794549634E-18,-0.0153,0.));
#47737=CARTESIAN_POINT('',(-0.00126635989804114,-0.0153,-1.55084359570465E-19));
#47738=CARTESIAN_POINT('Origin',(1.76941794549634E-18,-0.0153,0.));
#47739=CARTESIAN_POINT('Origin',(1.75785312232316E-18,-0.0152,0.));
#47740=CARTESIAN_POINT('Origin',(-0.00268445714771808,-0.0152,-3.28751185340118E-19));
#47741=CARTESIAN_POINT('Origin',(1.65376971376455E-18,-0.0143,0.));
#47742=CARTESIAN_POINT('',(-0.00116635989804114,-0.0144,-1.42837891578992E-19));
#47743=CARTESIAN_POINT('Origin',(1.66533453693773E-18,-0.0144,0.));
#47744=CARTESIAN_POINT('',(-0.00116635989804114,-0.0152,-1.42837891578992E-19));
#47745=CARTESIAN_POINT('',(-0.00116635989804114,-0.0143,-1.42837891578992E-19));
#47746=CARTESIAN_POINT('Origin',(1.75785312232316E-18,-0.0152,0.));
#47747=CARTESIAN_POINT('Origin',(1.65376971376455E-18,-0.0143,0.));
#47748=CARTESIAN_POINT('',(-0.00106635989804114,-0.0143,-1.30591423587518E-19));
#47749=CARTESIAN_POINT('Origin',(1.65376971376455E-18,-0.0143,0.));
#47750=CARTESIAN_POINT('Origin',(0.00900100000597247,-0.00900000021011351,
2.5166391089677E-7));
#47751=CARTESIAN_POINT('',(0.00900100000597247,-0.00900000021011351,0.00184504509674603));
#47752=CARTESIAN_POINT('Ctrl Pts',(-0.00380975858063243,-0.00899998937218426,
-0.00184137848958098));
#47753=CARTESIAN_POINT('Ctrl Pts',(-0.00380975858063243,-0.00893815389736155,
-0.00184159034836062));
#47754=CARTESIAN_POINT('Ctrl Pts',(-0.00380975858063243,-0.00887631623328271,
-0.00183865163430941));
#47755=CARTESIAN_POINT('Ctrl Pts',(-0.00380975858063243,-0.00881478413029403,
-0.00183246684420301));
#47756=CARTESIAN_POINT('Ctrl Pts',(-0.00353642309488705,-0.00858783002638803,
-0.00179790810359568));
#47757=CARTESIAN_POINT('Ctrl Pts',(-0.00353752250310302,-0.0086242637078,
-0.00180623272293779));
#47758=CARTESIAN_POINT('Ctrl Pts',(-0.00353849120739254,-0.00865990950754595,
-0.0018132613329253));
#47759=CARTESIAN_POINT('Ctrl Pts',(-0.00353932318339466,-0.00869447214609225,
-0.00181906562890172));
#47760=CARTESIAN_POINT('Ctrl Pts',(-0.00354192480978627,-0.00880255107189962,
-0.00183721592357208));
#47761=CARTESIAN_POINT('Ctrl Pts',(-0.00354318945087198,-0.00889995594775555,
-0.00184454176892423));
#47762=CARTESIAN_POINT('Ctrl Pts',(-0.00354320118263475,-0.00900000021011351,
-0.00184454176892423));
#47763=CARTESIAN_POINT('Origin',(0.00900100000597247,-0.00900000011651052,
3.82283508649252E-7));
#47764=CARTESIAN_POINT('',(-0.00380975858586299,-0.00900000011611844,-0.00134544337418665));
#47765=CARTESIAN_POINT('',(-0.00380975862800813,-0.00900000011337439,0.00134614011498439));
#47766=CARTESIAN_POINT('Origin',(-0.00380975860693448,-0.00899994566615699,
3.48370398817743E-7));
#47767=CARTESIAN_POINT('',(0.00900100000597247,-0.00900000011651052,0.00134621763185817));
#47768=CARTESIAN_POINT('',(-0.00337654510570282,-0.0084833905958057,-0.00124235155283125));
#47769=CARTESIAN_POINT('Ctrl Pts',(-0.00337620712303714,-0.00848339943917672,
-0.00124235522901977));
#47770=CARTESIAN_POINT('Ctrl Pts',(-0.00337756738494765,-0.00852772695862544,
-0.00126078198957128));
#47771=CARTESIAN_POINT('Ctrl Pts',(-0.0033788015330959,-0.00857301218210894,
-0.00127682532428018));
#47772=CARTESIAN_POINT('Ctrl Pts',(-0.00338003388768656,-0.00862570568134062,
-0.0012923761846553));
#47773=CARTESIAN_POINT('Ctrl Pts',(-0.00338018599196866,-0.00863236541625167,
-0.001294285824698));
#47774=CARTESIAN_POINT('Ctrl Pts',(-0.00338149651939755,-0.00869118133026391,
-0.00131066051706739));
#47775=CARTESIAN_POINT('Ctrl Pts',(-0.00338245034165808,-0.00874415513497043,
-0.00132201949741684));
#47776=CARTESIAN_POINT('Ctrl Pts',(-0.00338401193656355,-0.00886334276963602,
-0.00134014367932438));
#47777=CARTESIAN_POINT('Ctrl Pts',(-0.0033844896763387,-0.00892966491376065,
-0.00134525464698032));
#47778=CARTESIAN_POINT('Ctrl Pts',(-0.0033845085908206,-0.00899757065343684,
-0.00134545168095424));
#47779=CARTESIAN_POINT('Ctrl Pts',(-0.00338450877509932,-0.00899904621982914,
-0.00134545353568596));
#47780=CARTESIAN_POINT('Ctrl Pts',(-0.00338450873183093,-0.00900052178030331,
-0.00134545296373893));
#47781=CARTESIAN_POINT('Origin',(-0.00337226546574067,-0.00900117984349398,
2.58365129269925E-6));
#47782=CARTESIAN_POINT('Origin',(-0.00380975860693448,-0.00899994566615699,
3.48370398817743E-7));
#47783=CARTESIAN_POINT('Origin',(-0.00390975858063242,-0.00900003644744767,
0.0018421052628004));
#47784=CARTESIAN_POINT('',(-0.00390975858063242,-0.00900000344043453,-0.00174210526321707));
#47785=CARTESIAN_POINT('Ctrl Pts',(-0.00390975858063242,-0.00900000344043453,
-0.00174210526321707));
#47786=CARTESIAN_POINT('Ctrl Pts',(-0.00390975858063242,-0.00900010892359971,
-0.0017421052645996));
#47787=CARTESIAN_POINT('Ctrl Pts',(-0.00390975858063242,-0.00900021440675734,
-0.00174210525596106));
#47788=CARTESIAN_POINT('Ctrl Pts',(-0.00390975858063242,-0.0090003198899058,
-0.00174210523730213));
#47789=CARTESIAN_POINT('Ctrl Pts',(-0.00390975858063242,-0.00882510339125232,
-0.00173300347273605));
#47790=CARTESIAN_POINT('Ctrl Pts',(-0.00390975858063242,-0.00888321951194065,
-0.00173903303843893));
#47791=CARTESIAN_POINT('Ctrl Pts',(-0.00390975858063242,-0.00894161263180323,
-0.00174210449790967));
#47792=CARTESIAN_POINT('Ctrl Pts',(-0.00390975858063242,-0.00900000344043453,
-0.00174210526321707));
#47793=CARTESIAN_POINT('',(-0.00390966975442655,-0.00900000000006269,-0.00144210824574401));
#47794=CARTESIAN_POINT('',(-0.00390972476942416,-0.00799782182333048,-0.00104223077880221));
#47795=CARTESIAN_POINT('Ctrl Pts',(-0.00390966975442655,-0.00900000000006269,
-0.00144210824574401));
#47796=CARTESIAN_POINT('Ctrl Pts',(-0.00390966976203054,-0.0088197660211075,
-0.00144211226082542));
#47797=CARTESIAN_POINT('Ctrl Pts',(-0.0039096810567326,-0.00863964557616199,
-0.00140814906199155));
#47798=CARTESIAN_POINT('Ctrl Pts',(-0.00390969855902211,-0.00847221884979575,
-0.00134319471865232));
#47799=CARTESIAN_POINT('Ctrl Pts',(-0.0039097169364261,-0.0082964207871112,
-0.00127499265814613));
#47800=CARTESIAN_POINT('Ctrl Pts',(-0.00390972747686855,-0.00813461712028997,
-0.00117262355290227));
#47801=CARTESIAN_POINT('Ctrl Pts',(-0.00390972476942416,-0.00799782182333048,
-0.00104223077880221));
#47802=CARTESIAN_POINT('',(-0.00390971778425656,-0.00795392388178663,0.000998653228350628));
#47803=CARTESIAN_POINT('Ctrl Pts',(-0.00390972476942416,-0.00799782182333048,
-0.00104223077880221));
#47804=CARTESIAN_POINT('Ctrl Pts',(-0.00390972334479271,-0.00792584144088275,
-0.000973619342906699));
#47805=CARTESIAN_POINT('Ctrl Pts',(-0.00390972041610811,-0.0078607852822472,
-0.000897248810375659));
#47806=CARTESIAN_POINT('Ctrl Pts',(-0.0039097109017685,-0.00780438624911606,
-0.000815607003483071));
#47807=CARTESIAN_POINT('Ctrl Pts',(-0.00390970181578942,-0.00775052644847205,
-0.000737640925000353));
#47808=CARTESIAN_POINT('Ctrl Pts',(-0.00390968635523896,-0.0077045618950396,
-0.000654867542329328));
#47809=CARTESIAN_POINT('Ctrl Pts',(-0.00390967718883946,-0.00766715405430361,
-0.000567866545804131));
#47810=CARTESIAN_POINT('Ctrl Pts',(-0.00390966804404756,-0.00762983439362337,
-0.000481070633362192));
#47811=CARTESIAN_POINT('Ctrl Pts',(-0.00390966311664814,-0.00760103115841473,
-0.00039006693600034));
#47812=CARTESIAN_POINT('Ctrl Pts',(-0.00390965465336911,-0.00758136263727643,
-0.000297447048399321));
#47813=CARTESIAN_POINT('Ctrl Pts',(-0.00390964619108995,-0.00756169643980781,
-0.000204838103055954));
#47814=CARTESIAN_POINT('Ctrl Pts',(-0.00390963640198231,-0.00755116270600896,
-0.00011061345411514));
#47815=CARTESIAN_POINT('Ctrl Pts',(-0.00390963647383203,-0.00755009700252165,
-1.61629646556979E-5));
#47816=CARTESIAN_POINT('Ctrl Pts',(-0.00390963661393813,-0.00754801889331327,
0.000168014373805593));
#47817=CARTESIAN_POINT('Ctrl Pts',(-0.00390965471980009,-0.00758194386574754,
0.000353050874397227));
#47818=CARTESIAN_POINT('Ctrl Pts',(-0.00390967549689029,-0.00764941656405345,
0.000524809084816847));
#47819=CARTESIAN_POINT('Ctrl Pts',(-0.00390969678008587,-0.00771853281760433,
0.000700751122394549));
#47820=CARTESIAN_POINT('Ctrl Pts',(-0.00390971697562406,-0.00782285143124549,
0.000862759747474539));
#47821=CARTESIAN_POINT('Ctrl Pts',(-0.00390971778425656,-0.00795392388178663,
0.000998653228350628));
#47822=CARTESIAN_POINT('',(-0.00390963450991967,-0.00899994572134765,0.00144213270448328));
#47823=CARTESIAN_POINT('Ctrl Pts',(-0.00390971778425656,-0.00795392388178663,
0.000998653228350628));
#47824=CARTESIAN_POINT('Ctrl Pts',(-0.0039097185938505,-0.0080851521746966,
0.00113470828369855));
#47825=CARTESIAN_POINT('Ctrl Pts',(-0.00390970275420778,-0.00824319753023578,
0.00124458635119802));
#47826=CARTESIAN_POINT('Ctrl Pts',(-0.00390967849947921,-0.00841680717529352,
0.00132033545754371));
#47827=CARTESIAN_POINT('Ctrl Pts',(-0.00390965424331042,-0.00859042712900413,
0.00139608906174574));
#47828=CARTESIAN_POINT('Ctrl Pts',(-0.00390963265494929,-0.00877961385322806,
0.00143770908107385));
#47829=CARTESIAN_POINT('Ctrl Pts',(-0.00390963415795286,-0.00896918043380641,
0.00144179524960526));
#47830=CARTESIAN_POINT('Ctrl Pts',(-0.00390963423925692,-0.00897943492210449,
0.00144201628839417));
#47831=CARTESIAN_POINT('Ctrl Pts',(-0.00390963436154657,-0.00898969052073426,
0.00144212749742715));
#47832=CARTESIAN_POINT('Ctrl Pts',(-0.00390963450991967,-0.00899994572134765,
0.00144213270448328));
#47833=CARTESIAN_POINT('',(-0.00390971648405094,-0.0100016923901179,0.00104269314894275));
#47834=CARTESIAN_POINT('Ctrl Pts',(-0.00390963450991967,-0.00899994572134765,
0.00144213270448328));
#47835=CARTESIAN_POINT('Ctrl Pts',(-0.00390963735419761,-0.00917925816624089,
0.00144216106639203));
#47836=CARTESIAN_POINT('Ctrl Pts',(-0.00390965229205243,-0.00935824009674402,
0.00140874375267135));
#47837=CARTESIAN_POINT('Ctrl Pts',(-0.0039096719045267,-0.00952516270713903,
0.00134421182287322));
#47838=CARTESIAN_POINT('Ctrl Pts',(-0.00390969263859743,-0.00970163127318034,
0.00127598944671696));
#47839=CARTESIAN_POINT('Ctrl Pts',(-0.00390971467173984,-0.00986462208441464,
0.00117299239295296));
#47840=CARTESIAN_POINT('Ctrl Pts',(-0.00390971648405094,-0.0100016923901179,
0.00104269314894275));
#47841=CARTESIAN_POINT('',(-0.00390972211041965,-0.0100356073524843,-0.00100937059217969));
#47842=CARTESIAN_POINT('Ctrl Pts',(-0.00390971648405094,-0.0100016923901179,
0.00104269314894275));
#47843=CARTESIAN_POINT('Ctrl Pts',(-0.00390971829636204,-0.0101387626968384,
0.000912393903965479));
#47844=CARTESIAN_POINT('Ctrl Pts',(-0.0039097032843565,-0.0102499122404115,
0.000754792010601407));
#47845=CARTESIAN_POINT('Ctrl Pts',(-0.00390967824347019,-0.0103266137464934,
0.000582152223145582));
#47846=CARTESIAN_POINT('Ctrl Pts',(-0.00390965320258387,-0.0104033152526038,
0.00040951243562569));
#47847=CARTESIAN_POINT('Ctrl Pts',(-0.00390962578534569,-0.0104455689904412,
0.000221835420904369));
#47848=CARTESIAN_POINT('Ctrl Pts',(-0.00390963032251337,-0.0104496430802503,
3.218780127882E-5));
#47849=CARTESIAN_POINT('Ctrl Pts',(-0.0039096327045264,-0.0104517819774001,
-6.73771990263512E-5));
#47850=CARTESIAN_POINT('Ctrl Pts',(-0.00390964227984429,-0.0104433974606173,
-0.000167485522235034));
#47851=CARTESIAN_POINT('Ctrl Pts',(-0.00390964660722069,-0.0104250950124203,
-0.000265163779662066));
#47852=CARTESIAN_POINT('Ctrl Pts',(-0.00390965073883483,-0.0104076205321179,
-0.000358423258777086));
#47853=CARTESIAN_POINT('Ctrl Pts',(-0.00390965575216524,-0.0103811055941798,
-0.000449467563700001));
#47854=CARTESIAN_POINT('Ctrl Pts',(-0.00390966864830771,-0.0103455754734661,
-0.000537349171337576));
#47855=CARTESIAN_POINT('Ctrl Pts',(-0.00390968151389822,-0.0103101295263551,
-0.000625022580652821));
#47856=CARTESIAN_POINT('Ctrl Pts',(-0.00390969647605033,-0.0102657106427814,
-0.000709548144133988));
#47857=CARTESIAN_POINT('Ctrl Pts',(-0.00390970503051356,-0.0102136690684806,
-0.000788793353267544));
#47858=CARTESIAN_POINT('Ctrl Pts',(-0.00390971358396108,-0.0101616336733443,
-0.000868029153208667));
#47859=CARTESIAN_POINT('Ctrl Pts',(-0.00390971891000173,-0.0101019775683224,
-0.000941985919899507));
#47860=CARTESIAN_POINT('Ctrl Pts',(-0.00390972211041965,-0.0100356073524843,
-0.00100937059217969));
#47861=CARTESIAN_POINT('Ctrl Pts',(-0.00390972211041965,-0.0100356073524843,
-0.00100937059217969));
#47862=CARTESIAN_POINT('Ctrl Pts',(-0.0039097283511966,-0.00990618621974132,
-0.00114076990293808));
#47863=CARTESIAN_POINT('Ctrl Pts',(-0.00390971944756646,-0.00975123495878918,
-0.00124717904548944));
#47864=CARTESIAN_POINT('Ctrl Pts',(-0.00390970366359697,-0.00958177451303321,
-0.00132095260090437));
#47865=CARTESIAN_POINT('Ctrl Pts',(-0.00390968664417768,-0.00939904998466667,
-0.00140050059252555));
#47866=CARTESIAN_POINT('Ctrl Pts',(-0.00390966974601161,-0.00919945560991264,
-0.00144210380246136));
#47867=CARTESIAN_POINT('Ctrl Pts',(-0.00390966975442655,-0.00900000000006269,
-0.00144210824574401));
#47868=CARTESIAN_POINT('Origin',(0.,-0.009,-1.22464679914735E-19));
#47869=CARTESIAN_POINT('',(0.,-0.009,0.00125));
#47870=CARTESIAN_POINT('Origin',(0.,-0.009,-1.22464679914735E-19));
#47871=CARTESIAN_POINT('Origin',(-0.004,-0.009,-1.22464679914735E-19));
#47872=CARTESIAN_POINT('',(-0.004,-0.009,0.00125));
#47873=CARTESIAN_POINT('Ctrl Pts',(-0.00326780067323885,-0.00830775851653247,
-0.00103977630810674));
#47874=CARTESIAN_POINT('Ctrl Pts',(-0.00327714277681445,-0.00851186476585222,
-0.00117432822854541));
#47875=CARTESIAN_POINT('Ctrl Pts',(-0.0032846096979276,-0.0087559375999203,
-0.00124998758441102));
#47876=CARTESIAN_POINT('Ctrl Pts',(-0.00328461216640222,-0.00900000000000097,
-0.00124999998094225));
#47877=CARTESIAN_POINT('Ctrl Pts',(-0.00328461215845628,-0.00900048192889801,
-0.00124999990709781));
#47878=CARTESIAN_POINT('Ctrl Pts',(-0.00338400522957233,-0.00900048496365769,
-0.00124999990592778));
#47879=CARTESIAN_POINT('Ctrl Pts',(-0.00338461030538419,-0.00900052330173693,
-0.00134939112791716));
#47880=CARTESIAN_POINT('Ctrl Pts',(-0.00328462200345994,-0.0086739200473581,
-0.00125011657331827));
#47881=CARTESIAN_POINT('Ctrl Pts',(-0.003384013177488,-0.00867517913342947,
-0.00125011489397692));
#47882=CARTESIAN_POINT('Ctrl Pts',(-0.00338462023319443,-0.00864567411161468,
-0.00134951725455865));
#47883=CARTESIAN_POINT('Ctrl Pts',(-0.00325790117155621,-0.00802066659855702,
-0.000979447538677857));
#47884=CARTESIAN_POINT('Ctrl Pts',(-0.00336075013595249,-0.00800482732738064,
-0.000963468404288508));
#47885=CARTESIAN_POINT('Ctrl Pts',(-0.00335780888612222,-0.00793743054808474,
-0.00105840198561949));
#47886=CARTESIAN_POINT('Ctrl Pts',(-0.00321793190913946,-0.0076149676140644,
-1.54083867402206E-6));
#47887=CARTESIAN_POINT('Ctrl Pts',(-0.00332799412930291,-0.00761878655976351,
-1.51388930652299E-6));
#47888=CARTESIAN_POINT('Ctrl Pts',(-0.00331757760893123,-0.00749558137023603,
-1.66483058764779E-6));
#47889=CARTESIAN_POINT('Ctrl Pts',(-0.00325780785275684,-0.008019466089899,
0.000978742800856142));
#47890=CARTESIAN_POINT('Ctrl Pts',(-0.00336067162260847,-0.00800363754489395,
0.000962724449561964));
#47891=CARTESIAN_POINT('Ctrl Pts',(-0.0033577150665097,-0.00793612611646283,
0.0010576437152649));
#47892=CARTESIAN_POINT('Ctrl Pts',(-0.00329800025932114,-0.00899946420378033,
0.00138546387197374));
#47893=CARTESIAN_POINT('Ctrl Pts',(-0.0033953190356324,-0.00899944782531834,
0.00138926904137042));
#47894=CARTESIAN_POINT('Ctrl Pts',(-0.00339807408715874,-0.00899941917617344,
0.00149541593485778));
#47895=CARTESIAN_POINT('Ctrl Pts',(-0.00325786406347626,-0.00997987109426551,
0.000979401186339539));
#47896=CARTESIAN_POINT('Ctrl Pts',(-0.00336071891445555,-0.00999571441285378,
0.000963399852332962));
#47897=CARTESIAN_POINT('Ctrl Pts',(-0.00335777157893346,-0.010063153048397,
0.00105835340798998));
#47898=CARTESIAN_POINT('Ctrl Pts',(-0.00321793255865113,-0.0103850227343342,
-4.38299481707064E-7));
#47899=CARTESIAN_POINT('Ctrl Pts',(-0.00332799471446149,-0.0103812033852223,
-4.47410730017003E-7));
#47900=CARTESIAN_POINT('Ctrl Pts',(-0.00331757825861524,-0.0105044081817788,
-4.72359875001561E-7));
#47901=CARTESIAN_POINT('Ctrl Pts',(-0.00325784210153424,-0.00998003788779652,
-0.000978747541355083));
#47902=CARTESIAN_POINT('Ctrl Pts',(-0.00336070043689,-0.00999586177973733,
-0.00096275163289535));
#47903=CARTESIAN_POINT('Ctrl Pts',(-0.00335774949912804,-0.0100633355839779,
-0.00105764734367712));
#47904=CARTESIAN_POINT('Ctrl Pts',(-0.00328460231345262,-0.00932704381043793,
-0.00124988324087735));
#47905=CARTESIAN_POINT('Ctrl Pts',(-0.00338399728153908,-0.00932579560598706,
-0.00124988491617768));
#47906=CARTESIAN_POINT('Ctrl Pts',(-0.00338460037758513,-0.00935537209178598,
-0.00134926500141788));
#47907=CARTESIAN_POINT('Ctrl Pts',(-0.00328461215845628,-0.00900048192889801,
-0.00124999990709781));
#47908=CARTESIAN_POINT('Ctrl Pts',(-0.00338400522957233,-0.00900048496365769,
-0.00124999990592778));
#47909=CARTESIAN_POINT('Ctrl Pts',(-0.00338461030538419,-0.00900052330173693,
-0.00134939112791716));
#47910=CARTESIAN_POINT('Ctrl Pts',(-0.0035392791351489,-0.00858849912814965,
-0.00179466521288696));
#47911=CARTESIAN_POINT('Ctrl Pts',(-0.00342573153923465,-0.00859176400850957,
-0.00179333404984997));
#47912=CARTESIAN_POINT('Ctrl Pts',(-0.00343811948343117,-0.00856602524158671,
-0.00190328650635992));
#47913=CARTESIAN_POINT('Ctrl Pts',(-0.00355142559943888,-0.00905859136078448,
-0.00190144952999438));
#47914=CARTESIAN_POINT('Ctrl Pts',(-0.00343722171108695,-0.00906840205799737,
-0.00190374929419889));
#47915=CARTESIAN_POINT('Ctrl Pts',(-0.0034503400565124,-0.00906157284819796,
-0.0020166590821151));
#47916=CARTESIAN_POINT('Ctrl Pts',(-0.00352537010396588,-0.0100884377158575,
-0.00172789987787408));
#47917=CARTESIAN_POINT('Ctrl Pts',(-0.0034151603753512,-0.0100497091309754,
-0.00174559426658833));
#47918=CARTESIAN_POINT('Ctrl Pts',(-0.00342416641781692,-0.0101460057925454,
-0.00183316467220812));
#47919=CARTESIAN_POINT('Ctrl Pts',(-0.00341335748290235,-0.0109970962519671,
-0.000457281663563109));
#47920=CARTESIAN_POINT('Ctrl Pts',(-0.00331425963473675,-0.010996887331939,
-0.000476856829642387));
#47921=CARTESIAN_POINT('Ctrl Pts',(-0.0033115684832145,-0.0111050748119872,
-0.000486036946141634));
#47922=CARTESIAN_POINT('Ctrl Pts',(-0.00345233946123927,-0.0107338060170907,
0.00108652455487473));
#47923=CARTESIAN_POINT('Ctrl Pts',(-0.00335032457735252,-0.0107129565277369,
0.00112100474052161));
#47924=CARTESIAN_POINT('Ctrl Pts',(-0.00335076613415529,-0.0108274712600009,
0.00115282043607336));
#47925=CARTESIAN_POINT('Ctrl Pts',(-0.00356449374860163,-0.00945621932640169,
0.00198829625682747));
#47926=CARTESIAN_POINT('Ctrl Pts',(-0.00344854884364189,-0.00943365667565594,
0.00198475236629158));
#47927=CARTESIAN_POINT('Ctrl Pts',(-0.0034634722557383,-0.00948068538942303,
0.00210854197031486));
#47928=CARTESIAN_POINT('Ctrl Pts',(-0.00352531374816938,-0.00791032423527775,
0.00172792526671951));
#47929=CARTESIAN_POINT('Ctrl Pts',(-0.00341511348123987,-0.00794907951679388,
0.00174568140804206));
#47930=CARTESIAN_POINT('Ctrl Pts',(-0.00342410980697788,-0.0078526998577211,
0.00183315731298699));
#47931=CARTESIAN_POINT('Ctrl Pts',(-0.00341328178572483,-0.00700287546046352,
0.000454633913679566));
#47932=CARTESIAN_POINT('Ctrl Pts',(-0.00331419107940177,-0.00700305969526376,
0.000474177195847323));
#47933=CARTESIAN_POINT('Ctrl Pts',(-0.00331149240063511,-0.00689487285927746,
0.000483300740605997));
#47934=CARTESIAN_POINT('Ctrl Pts',(-0.00345241595160808,-0.00726632486312327,
-0.00108656836792835));
#47935=CARTESIAN_POINT('Ctrl Pts',(-0.00335038976344317,-0.00728717254733531,
-0.00112102914438496));
#47936=CARTESIAN_POINT('Ctrl Pts',(-0.00335084297932956,-0.00717272015287796,
-0.00115292921767708));
#47937=CARTESIAN_POINT('Ctrl Pts',(-0.00352712997637068,-0.00811830261348138,
-0.00168785720747976));
#47938=CARTESIAN_POINT('Ctrl Pts',(-0.00341440081056064,-0.00812174001897434,
-0.00168445098079964));
#47939=CARTESIAN_POINT('Ctrl Pts',(-0.00342589891034995,-0.00807047763497546,
-0.00178991393060475));
#47940=CARTESIAN_POINT('Ctrl Pts',(-0.0035392791351489,-0.00858849912814965,
-0.00179466521288696));
#47941=CARTESIAN_POINT('Ctrl Pts',(-0.00342573153923465,-0.00859176400850957,
-0.00179333404984997));
#47942=CARTESIAN_POINT('Ctrl Pts',(-0.00343811948343117,-0.00856602524158671,
-0.00190328650635992));
#47943=CARTESIAN_POINT('Origin',(-0.00380969939533716,-0.00899994566562597,
3.48367311799158E-7));
#47944=CARTESIAN_POINT('Origin',(-0.00380969419167622,-0.00899994566562597,
0.00144616158862221));
#47945=CARTESIAN_POINT('Ctrl Pts',(-0.00380975858063242,-0.00881478413029403,
-0.00183246684420301));
#47946=CARTESIAN_POINT('Ctrl Pts',(-0.00390993294014545,-0.00881478413029403,
-0.00183246684420301));
#47947=CARTESIAN_POINT('Ctrl Pts',(-0.00390975842889103,-0.00882512165273333,
-0.00173282745701358));
#47948=CARTESIAN_POINT('Ctrl Pts',(-0.00380975858063242,-0.00929465142715738,
-0.0018806998537358));
#47949=CARTESIAN_POINT('Ctrl Pts',(-0.00390993294014545,-0.00929465142715738,
-0.0018806998537358));
#47950=CARTESIAN_POINT('Ctrl Pts',(-0.00390975842889103,-0.00927906675289324,
-0.00177836203380147));
#47951=CARTESIAN_POINT('Ctrl Pts',(-0.00380975858063242,-0.0102936387094841,
-0.00158253456509613));
#47952=CARTESIAN_POINT('Ctrl Pts',(-0.00390993294014546,-0.0102936387094841,
-0.00158253456509614));
#47953=CARTESIAN_POINT('Ctrl Pts',(-0.00390975842889104,-0.0102241270617854,
-0.00149607241763065));
#47954=CARTESIAN_POINT('Ctrl Pts',(-0.00380975858063242,-0.0110403459009329,
-0.000207601983482724));
#47955=CARTESIAN_POINT('Ctrl Pts',(-0.00390993294014544,-0.0110403459009329,
-0.000207601983482722));
#47956=CARTESIAN_POINT('Ctrl Pts',(-0.00390975842889102,-0.0109298209858678,
-0.00019577210929604));
#47957=CARTESIAN_POINT('Ctrl Pts',(-0.00380975858063243,-0.010585488822892,
0.00129440175744357));
#47958=CARTESIAN_POINT('Ctrl Pts',(-0.00390993294014546,-0.010585488822892,
0.00129440175744357));
#47959=CARTESIAN_POINT('Ctrl Pts',(-0.00390975842889104,-0.0104994209642949,
0.0012241417666484));
#47960=CARTESIAN_POINT('Ctrl Pts',(-0.00380975858063242,-0.00920314460986179,
0.00202990873817867));
#47961=CARTESIAN_POINT('Ctrl Pts',(-0.00390993294014544,-0.00920314460986179,
0.00202990873817867));
#47962=CARTESIAN_POINT('Ctrl Pts',(-0.00390975842889102,-0.00919187984963056,
0.00191958960744435));
#47963=CARTESIAN_POINT('Ctrl Pts',(-0.00380975858063242,-0.00770446035061261,
0.0015817160659287));
#47964=CARTESIAN_POINT('Ctrl Pts',(-0.00390993294014545,-0.00770446035061261,
0.0015817160659287));
#47965=CARTESIAN_POINT('Ctrl Pts',(-0.00390975842889103,-0.00777409310458325,
0.00149536140507255));
#47966=CARTESIAN_POINT('Ctrl Pts',(-0.00380975858063242,-0.00695993177951074,
0.000203870131802003));
#47967=CARTESIAN_POINT('Ctrl Pts',(-0.00390993294014545,-0.00695993177951073,
0.000203870131802006));
#47968=CARTESIAN_POINT('Ctrl Pts',(-0.00390975842889103,-0.00707045087524681,
0.000192132115288156));
#47969=CARTESIAN_POINT('Ctrl Pts',(-0.00380975858063242,-0.00741443492830406,
-0.00129313650789938));
#47970=CARTESIAN_POINT('Ctrl Pts',(-0.00390993294014545,-0.00741443492830407,
-0.00129313650789939));
#47971=CARTESIAN_POINT('Ctrl Pts',(-0.00390975842889103,-0.00750045646082591,
-0.00122286495690331));
#47972=CARTESIAN_POINT('Ctrl Pts',(-0.00380975858063242,-0.00833491683343068,
-0.00178423383467021));
#47973=CARTESIAN_POINT('Ctrl Pts',(-0.00390993294014545,-0.00833491683343068,
-0.00178423383467021));
#47974=CARTESIAN_POINT('Ctrl Pts',(-0.00390975842889103,-0.00837117655257341,
-0.00168729288022569));
#47975=CARTESIAN_POINT('Ctrl Pts',(-0.00380975858063242,-0.00881478413029403,
-0.00183246684420301));
#47976=CARTESIAN_POINT('Ctrl Pts',(-0.00390993294014545,-0.00881478413029403,
-0.00183246684420301));
#47977=CARTESIAN_POINT('Ctrl Pts',(-0.00390975842889103,-0.00882512165273333,
-0.00173282745701358));
#47978=CARTESIAN_POINT('Origin',(1.66533453693773E-18,-0.0144,0.));
#47979=CARTESIAN_POINT('Origin',(-0.00106635989804114,-0.0144,-1.30591423587518E-19));
#47980=CARTESIAN_POINT('Origin',(1.75785312232316E-18,-0.0152,0.));
#47981=CARTESIAN_POINT('Origin',(-0.00126635989804114,-0.0152,-1.55084359570465E-19));
#47982=CARTESIAN_POINT('Origin',(-1.86727542905182E-18,0.014,0.));
#47983=CARTESIAN_POINT('Origin',(0.0045,0.014,-5.51091059616309E-19));
#54554=UNCERTAINTY_MEASURE_WITH_UNIT(LENGTH_MEASURE(1.E-5),#54581,
'DISTANCE_ACCURACY_VALUE',
'Maximum model space distance between geometric entities at asserted c
onnectivities');
#54564=UNCERTAINTY_MEASURE_WITH_UNIT(LENGTH_MEASURE(1.E-5),#54581,
'DISTANCE_ACCURACY_VALUE',
'Maximum model space distance between geometric entities at asserted c
onnectivities');
#54570=(
GEOMETRIC_REPRESENTATION_CONTEXT(3)
GLOBAL_UNCERTAINTY_ASSIGNED_CONTEXT((#54554))
GLOBAL_UNIT_ASSIGNED_CONTEXT((#54581,#54582,#54583))
REPRESENTATION_CONTEXT('','3D')
);
#54580=(
GEOMETRIC_REPRESENTATION_CONTEXT(3)
GLOBAL_UNCERTAINTY_ASSIGNED_CONTEXT((#54564))
GLOBAL_UNIT_ASSIGNED_CONTEXT((#54581,#54582,#54583))
REPRESENTATION_CONTEXT('','3D')
);
#54581=(
LENGTH_UNIT()
NAMED_UNIT(*)
SI_UNIT($,.METRE.)
);
#54582=(
NAMED_UNIT(*)
PLANE_ANGLE_UNIT()
SI_UNIT($,.RADIAN.)
);
#54583=(
NAMED_UNIT(*)
SI_UNIT($,.STERADIAN.)
SOLID_ANGLE_UNIT()
);
#54589=SHAPE_DEFINITION_REPRESENTATION(#54604,#54634);
#54604=PRODUCT_DEFINITION_SHAPE('',$,#54650);
#54634=SHAPE_REPRESENTATION('',(#18747),#54570);
#54644=PRODUCT_DEFINITION_CONTEXT('part definition',#54691,'design');
#54650=PRODUCT_DEFINITION('sockethead','Sockethead',#54665,#54644);
#54665=PRODUCT_DEFINITION_FORMATION('',$,#54698);
#54691=APPLICATION_CONTEXT(
'Core Data for Automotive Mechanical Design Process');
#54692=PRODUCT_CONTEXT('part definition',#54691,'mechanical');
#54698=PRODUCT('sockethead','Sockethead','sockethead',(#54692));
#54709=PRESENTATION_STYLE_ASSIGNMENT((#54719));
#54713=PRESENTATION_STYLE_ASSIGNMENT((#54723));
#54715=PRESENTATION_STYLE_ASSIGNMENT((#54725));
#54719=SURFACE_STYLE_USAGE(.BOTH.,#54729);
#54723=SURFACE_STYLE_USAGE(.BOTH.,#54733);
#54725=SURFACE_STYLE_USAGE(.BOTH.,#54735);
#54729=SURFACE_SIDE_STYLE('',(#54739));
#54733=SURFACE_SIDE_STYLE('',(#54743));
#54735=SURFACE_SIDE_STYLE('',(#54745));
#54739=SURFACE_STYLE_FILL_AREA(#54749);
#54743=SURFACE_STYLE_FILL_AREA(#54753);
#54745=SURFACE_STYLE_FILL_AREA(#54755);
#54749=FILL_AREA_STYLE('Opaque(153,153,153)',(#54759));
#54753=FILL_AREA_STYLE('Opaque(163,170,173)',(#54763));
#54755=FILL_AREA_STYLE('Opaque(15,15,15)',(#54765));
#54759=FILL_AREA_STYLE_COLOUR('Opaque(153,153,153)',#54769);
#54763=FILL_AREA_STYLE_COLOUR('Opaque(163,170,173)',#54773);
#54765=FILL_AREA_STYLE_COLOUR('Opaque(15,15,15)',#54775);
#54769=COLOUR_RGB('Opaque(153,153,153)', 0.09019608, 0.27058824, 0.51372549);
#54773=COLOUR_RGB('Opaque(163,170,173)', 0.31764706, 0.68627451, 0.89019608);
#54775=COLOUR_RGB('Opaque(15,15,15)', 0.72549020, 0.75294118, 0.79215686);
ENDSEC;
END-ISO-10303-21;
